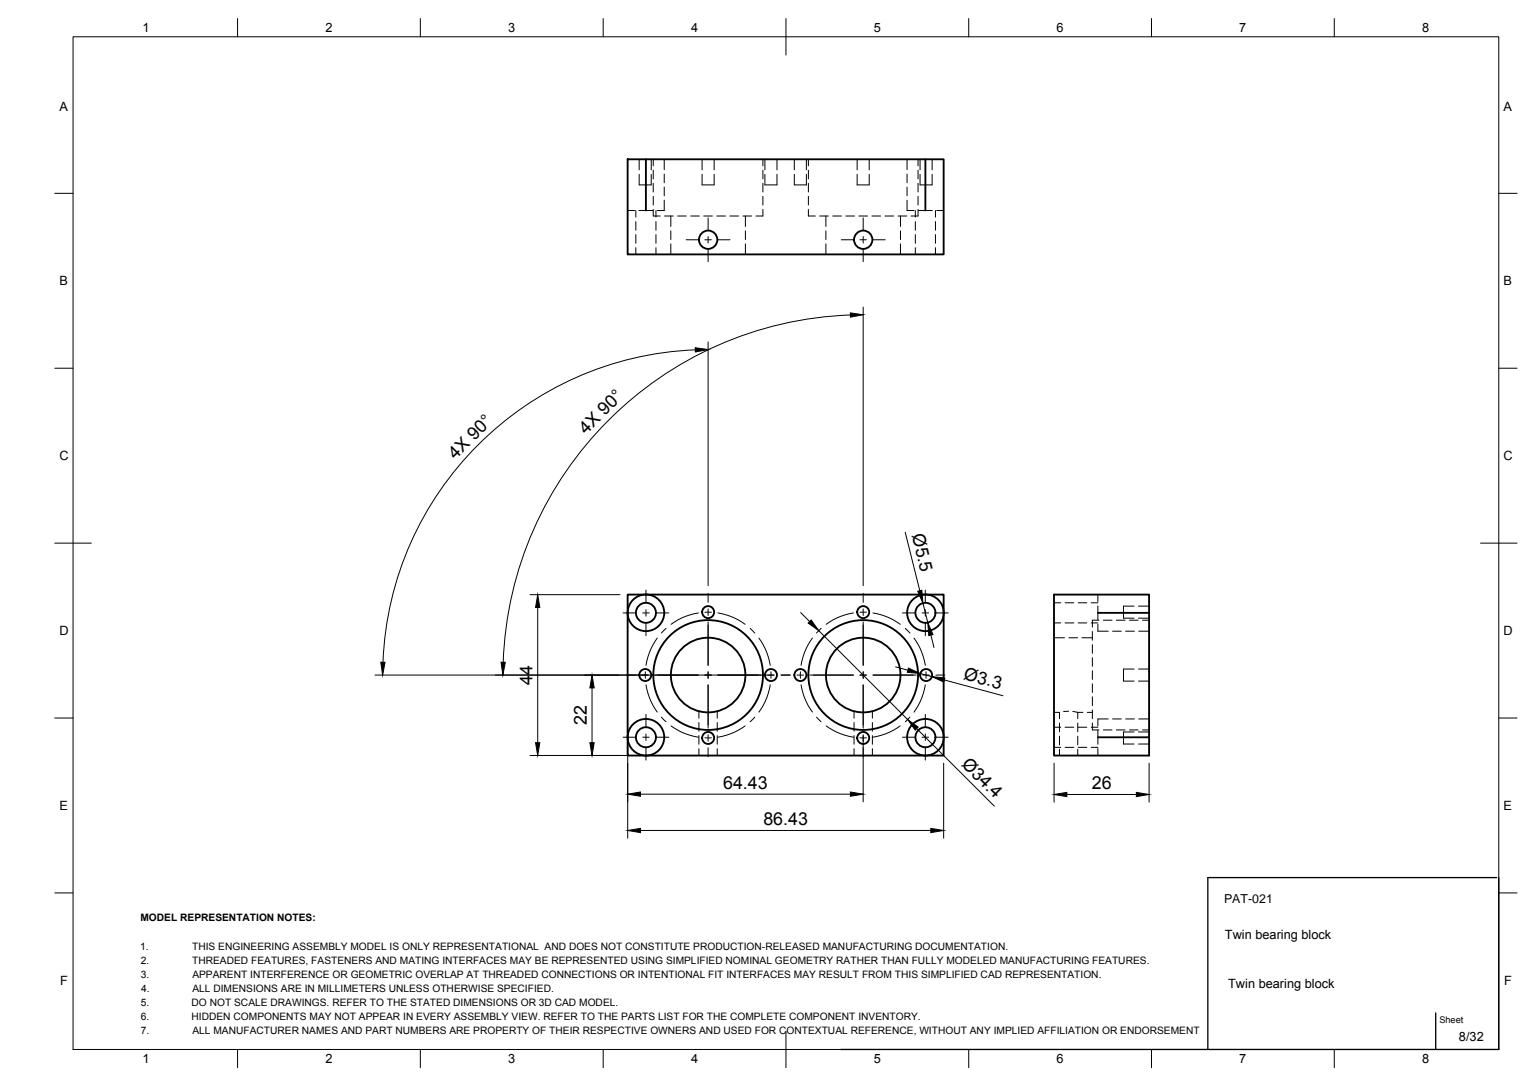
ISO-10303-21;
HEADER;
/* Generated by software containing ST-Developer
 * from STEP Tools, Inc. (www.steptools.com) 
 */

FILE_DESCRIPTION(
/* description */ ('Chain-less indexing wheel (Geneva) drive'),
/* implementation_level */ '2;1');

FILE_NAME(
/* name */ 'Twin bearing block.step',
/* time_stamp */ '2026-10-28T03:25:22-07:00',
/* author */ (''),
/* organization */ (''),
/* preprocessor_version */ 'ST-DEVELOPER v20.2',
/* originating_system */ 'Autodesk Translation Framework v15.17.0.0',
/* authorisation */ '');

FILE_SCHEMA (('AUTOMOTIVE_DESIGN { 1 0 10303 214 3 1 1 }'));
ENDSEC;

DATA;
#10=MECHANICAL_DESIGN_GEOMETRIC_PRESENTATION_REPRESENTATION('',(#306),#10957);
#213=B_SPLINE_CURVE_WITH_KNOTS('',3,(#8714,#8715,#8716,#8717,#8718,#8719,
#8720,#8721,#8722,#8723,#8724,#8725,#8726,#8727,#8728,#8729,#8730,#8731,
#8732,#8733,#8734,#8735,#8736,#8737,#8738,#8739,#8740,#8741,#8742,#8743,
#8744,#8745,#8746,#8747),.UNSPECIFIED.,.T.,.F.,(4,2,2,2,2,2,2,2,2,2,2,2,
2,2,2,2,4),(0.,0.094594182476448,0.189188364952896,0.283770357603024,0.378352350253152,
0.472934342903279,0.567516335553407,0.662110518029855,0.756704700506303,
0.851298882982751,0.945893065459199,1.04047505810933,1.13505705075945,1.22963904340958,
1.32422103605971,1.41881521853616,1.51340940101261),.UNSPECIFIED.);
#214=B_SPLINE_CURVE_WITH_KNOTS('',3,(#8794,#8795,#8796,#8797,#8798,#8799,
#8800,#8801,#8802,#8803,#8804,#8805,#8806,#8807,#8808,#8809,#8810,#8811,
#8812,#8813,#8814,#8815,#8816,#8817,#8818,#8819,#8820,#8821,#8822,#8823,
#8824,#8825,#8826,#8827),.UNSPECIFIED.,.T.,.F.,(4,2,2,2,2,2,2,2,2,2,2,2,
2,2,2,2,4),(0.,0.0945941824764479,0.189188364952896,0.283770357603024,0.378352350253152,
0.47293434290328,0.567516335553408,0.662110518029856,0.756704700506303,
0.851298882982751,0.945893065459199,1.04047505810933,1.13505705075946,1.22963904340958,
1.32422103605971,1.41881521853616,1.51340940101261),.UNSPECIFIED.);
#256=SHAPE_REPRESENTATION_RELATIONSHIP('SRR','None',#11069,#281);
#281=ADVANCED_BREP_SHAPE_REPRESENTATION('',(#339),#10932);
#306=STYLED_ITEM('',(#11287),#339);
#339=MANIFOLD_SOLID_BREP('Body1',#5702);
#375=FACE_BOUND('',#1026,.T.);
#376=FACE_BOUND('',#1028,.T.);
#377=FACE_BOUND('',#1040,.T.);
#378=FACE_BOUND('',#1042,.T.);
#379=FACE_BOUND('',#1046,.T.);
#380=FACE_BOUND('',#1050,.T.);
#381=FACE_BOUND('',#1054,.T.);
#382=FACE_BOUND('',#1058,.T.);
#383=FACE_BOUND('',#1063,.T.);
#384=FACE_BOUND('',#1064,.T.);
#385=FACE_BOUND('',#1065,.T.);
#386=FACE_BOUND('',#1066,.T.);
#387=FACE_BOUND('',#1067,.T.);
#388=FACE_BOUND('',#1068,.T.);
#389=FACE_BOUND('',#1069,.T.);
#390=FACE_BOUND('',#1070,.T.);
#391=FACE_BOUND('',#1071,.T.);
#392=FACE_BOUND('',#1072,.T.);
#393=FACE_BOUND('',#1081,.T.);
#394=FACE_BOUND('',#1082,.T.);
#395=FACE_BOUND('',#1085,.T.);
#396=FACE_BOUND('',#1086,.T.);
#397=FACE_BOUND('',#1087,.T.);
#398=FACE_BOUND('',#1088,.T.);
#399=FACE_BOUND('',#1089,.T.);
#400=FACE_BOUND('',#1090,.T.);
#490=PLANE('',#6051);
#491=PLANE('',#6055);
#492=PLANE('',#6059);
#493=PLANE('',#6063);
#494=PLANE('',#6067);
#495=PLANE('',#6076);
#496=PLANE('',#6080);
#497=PLANE('',#6084);
#498=PLANE('',#6088);
#499=PLANE('',#6092);
#500=PLANE('',#6102);
#501=PLANE('',#6110);
#502=PLANE('',#6118);
#503=PLANE('',#6126);
#504=PLANE('',#6128);
#505=PLANE('',#6129);
#506=PLANE('',#6130);
#507=PLANE('',#6131);
#508=PLANE('',#6132);
#509=PLANE('',#6141);
#510=PLANE('',#6142);
#511=PLANE('',#6143);
#512=PLANE('',#6144);
#513=PLANE('',#6145);
#674=FACE_OUTER_BOUND('',#1015,.T.);
#675=FACE_OUTER_BOUND('',#1016,.T.);
#676=FACE_OUTER_BOUND('',#1017,.T.);
#677=FACE_OUTER_BOUND('',#1018,.T.);
#678=FACE_OUTER_BOUND('',#1019,.T.);
#679=FACE_OUTER_BOUND('',#1020,.T.);
#680=FACE_OUTER_BOUND('',#1021,.T.);
#681=FACE_OUTER_BOUND('',#1022,.T.);
#682=FACE_OUTER_BOUND('',#1023,.T.);
#683=FACE_OUTER_BOUND('',#1024,.T.);
#684=FACE_OUTER_BOUND('',#1025,.T.);
#685=FACE_OUTER_BOUND('',#1027,.T.);
#686=FACE_OUTER_BOUND('',#1029,.T.);
#687=FACE_OUTER_BOUND('',#1030,.T.);
#688=FACE_OUTER_BOUND('',#1031,.T.);
#689=FACE_OUTER_BOUND('',#1032,.T.);
#690=FACE_OUTER_BOUND('',#1033,.T.);
#691=FACE_OUTER_BOUND('',#1034,.T.);
#692=FACE_OUTER_BOUND('',#1035,.T.);
#693=FACE_OUTER_BOUND('',#1036,.T.);
#694=FACE_OUTER_BOUND('',#1037,.T.);
#695=FACE_OUTER_BOUND('',#1038,.T.);
#696=FACE_OUTER_BOUND('',#1039,.T.);
#697=FACE_OUTER_BOUND('',#1041,.T.);
#698=FACE_OUTER_BOUND('',#1043,.T.);
#699=FACE_OUTER_BOUND('',#1044,.T.);
#700=FACE_OUTER_BOUND('',#1045,.T.);
#701=FACE_OUTER_BOUND('',#1047,.T.);
#702=FACE_OUTER_BOUND('',#1048,.T.);
#703=FACE_OUTER_BOUND('',#1049,.T.);
#704=FACE_OUTER_BOUND('',#1051,.T.);
#705=FACE_OUTER_BOUND('',#1052,.T.);
#706=FACE_OUTER_BOUND('',#1053,.T.);
#707=FACE_OUTER_BOUND('',#1055,.T.);
#708=FACE_OUTER_BOUND('',#1056,.T.);
#709=FACE_OUTER_BOUND('',#1057,.T.);
#710=FACE_OUTER_BOUND('',#1059,.T.);
#711=FACE_OUTER_BOUND('',#1060,.T.);
#712=FACE_OUTER_BOUND('',#1061,.T.);
#713=FACE_OUTER_BOUND('',#1062,.T.);
#714=FACE_OUTER_BOUND('',#1073,.T.);
#715=FACE_OUTER_BOUND('',#1074,.T.);
#716=FACE_OUTER_BOUND('',#1075,.T.);
#717=FACE_OUTER_BOUND('',#1076,.T.);
#718=FACE_OUTER_BOUND('',#1077,.T.);
#719=FACE_OUTER_BOUND('',#1078,.T.);
#720=FACE_OUTER_BOUND('',#1079,.T.);
#721=FACE_OUTER_BOUND('',#1080,.T.);
#722=FACE_OUTER_BOUND('',#1083,.T.);
#723=FACE_OUTER_BOUND('',#1084,.T.);
#1015=EDGE_LOOP('',(#3843,#3844,#3845,#3846));
#1016=EDGE_LOOP('',(#3847,#3848,#3849,#3850));
#1017=EDGE_LOOP('',(#3851));
#1018=EDGE_LOOP('',(#3852,#3853,#3854,#3855));
#1019=EDGE_LOOP('',(#3856));
#1020=EDGE_LOOP('',(#3857,#3858,#3859,#3860));
#1021=EDGE_LOOP('',(#3861));
#1022=EDGE_LOOP('',(#3862,#3863,#3864,#3865));
#1023=EDGE_LOOP('',(#3866));
#1024=EDGE_LOOP('',(#3867,#3868,#3869,#3870));
#1025=EDGE_LOOP('',(#3871));
#1026=EDGE_LOOP('',(#3872));
#1027=EDGE_LOOP('',(#3873,#3874,#3875,#3876));
#1028=EDGE_LOOP('',(#3877));
#1029=EDGE_LOOP('',(#3878,#3879,#3880,#3881));
#1030=EDGE_LOOP('',(#3882,#3883,#3884,#3885));
#1031=EDGE_LOOP('',(#3886));
#1032=EDGE_LOOP('',(#3887,#3888,#3889,#3890));
#1033=EDGE_LOOP('',(#3891));
#1034=EDGE_LOOP('',(#3892,#3893,#3894,#3895));
#1035=EDGE_LOOP('',(#3896));
#1036=EDGE_LOOP('',(#3897,#3898,#3899,#3900));
#1037=EDGE_LOOP('',(#3901));
#1038=EDGE_LOOP('',(#3902,#3903,#3904,#3905));
#1039=EDGE_LOOP('',(#3906));
#1040=EDGE_LOOP('',(#3907));
#1041=EDGE_LOOP('',(#3908,#3909,#3910,#3911));
#1042=EDGE_LOOP('',(#3912));
#1043=EDGE_LOOP('',(#3913,#3914,#3915,#3916));
#1044=EDGE_LOOP('',(#3917,#3918,#3919,#3920));
#1045=EDGE_LOOP('',(#3921,#3922));
#1046=EDGE_LOOP('',(#3923));
#1047=EDGE_LOOP('',(#3924,#3925,#3926,#3927));
#1048=EDGE_LOOP('',(#3928,#3929,#3930,#3931));
#1049=EDGE_LOOP('',(#3932,#3933));
#1050=EDGE_LOOP('',(#3934));
#1051=EDGE_LOOP('',(#3935,#3936,#3937,#3938));
#1052=EDGE_LOOP('',(#3939,#3940,#3941,#3942));
#1053=EDGE_LOOP('',(#3943,#3944));
#1054=EDGE_LOOP('',(#3945));
#1055=EDGE_LOOP('',(#3946,#3947,#3948,#3949));
#1056=EDGE_LOOP('',(#3950,#3951,#3952,#3953));
#1057=EDGE_LOOP('',(#3954,#3955));
#1058=EDGE_LOOP('',(#3956));
#1059=EDGE_LOOP('',(#3957,#3958,#3959));
#1060=EDGE_LOOP('',(#3960,#3961,#3962));
#1061=EDGE_LOOP('',(#3963,#3964,#3965));
#1062=EDGE_LOOP('',(#3966,#3967,#3968,#3969,#3970,#3971,#3972,#3973));
#1063=EDGE_LOOP('',(#3974));
#1064=EDGE_LOOP('',(#3975));
#1065=EDGE_LOOP('',(#3976));
#1066=EDGE_LOOP('',(#3977));
#1067=EDGE_LOOP('',(#3978));
#1068=EDGE_LOOP('',(#3979));
#1069=EDGE_LOOP('',(#3980));
#1070=EDGE_LOOP('',(#3981));
#1071=EDGE_LOOP('',(#3982));
#1072=EDGE_LOOP('',(#3983));
#1073=EDGE_LOOP('',(#3984,#3985,#3986));
#1074=EDGE_LOOP('',(#3987,#3988,#3989,#3990));
#1075=EDGE_LOOP('',(#3991,#3992,#3993,#3994));
#1076=EDGE_LOOP('',(#3995,#3996,#3997,#3998));
#1077=EDGE_LOOP('',(#3999,#4000,#4001,#4002));
#1078=EDGE_LOOP('',(#4003,#4004,#4005,#4006,#4007,#4008,#4009,#4010,#4011,
#4012));
#1079=EDGE_LOOP('',(#4013,#4014,#4015,#4016,#4017,#4018,#4019,#4020,#4021,
#4022));
#1080=EDGE_LOOP('',(#4023,#4024,#4025,#4026,#4027,#4028,#4029,#4030,#4031,
#4032));
#1081=EDGE_LOOP('',(#4033));
#1082=EDGE_LOOP('',(#4034));
#1083=EDGE_LOOP('',(#4035,#4036,#4037,#4038,#4039,#4040,#4041,#4042,#4043,
#4044));
#1084=EDGE_LOOP('',(#4045,#4046,#4047,#4048));
#1085=EDGE_LOOP('',(#4049));
#1086=EDGE_LOOP('',(#4050));
#1087=EDGE_LOOP('',(#4051));
#1088=EDGE_LOOP('',(#4052));
#1089=EDGE_LOOP('',(#4053));
#1090=EDGE_LOOP('',(#4054));
#1463=LINE('',#8713,#1837);
#1464=LINE('',#8752,#1838);
#1465=LINE('',#8759,#1839);
#1466=LINE('',#8766,#1840);
#1467=LINE('',#8773,#1841);
#1468=LINE('',#8780,#1842);
#1469=LINE('',#8788,#1843);
#1470=LINE('',#8793,#1844);
#1471=LINE('',#8832,#1845);
#1472=LINE('',#8839,#1846);
#1473=LINE('',#8846,#1847);
#1474=LINE('',#8853,#1848);
#1475=LINE('',#8860,#1849);
#1476=LINE('',#8868,#1850);
#1477=LINE('',#8872,#1851);
#1478=LINE('',#8876,#1852);
#1479=LINE('',#8879,#1853);
#1480=LINE('',#8881,#1854);
#1481=LINE('',#8889,#1855);
#1482=LINE('',#8893,#1856);
#1483=LINE('',#8896,#1857);
#1484=LINE('',#8898,#1858);
#1485=LINE('',#8906,#1859);
#1486=LINE('',#8910,#1860);
#1487=LINE('',#8913,#1861);
#1488=LINE('',#8915,#1862);
#1489=LINE('',#8923,#1863);
#1490=LINE('',#8927,#1864);
#1491=LINE('',#8930,#1865);
#1492=LINE('',#8932,#1866);
#1493=LINE('',#8939,#1867);
#1494=LINE('',#8940,#1868);
#1495=LINE('',#8943,#1869);
#1496=LINE('',#8944,#1870);
#1497=LINE('',#8947,#1871);
#1498=LINE('',#8948,#1872);
#1499=LINE('',#8950,#1873);
#1500=LINE('',#8951,#1874);
#1501=LINE('',#8952,#1875);
#1502=LINE('',#8953,#1876);
#1503=LINE('',#8956,#1877);
#1504=LINE('',#8957,#1878);
#1505=LINE('',#8961,#1879);
#1506=LINE('',#8965,#1880);
#1507=LINE('',#8969,#1881);
#1508=LINE('',#8973,#1882);
#1509=LINE('',#8977,#1883);
#1510=LINE('',#8978,#1884);
#1511=LINE('',#8979,#1885);
#1512=LINE('',#8982,#1886);
#1513=LINE('',#8983,#1887);
#1514=LINE('',#8986,#1888);
#1515=LINE('',#8987,#1889);
#1516=LINE('',#8989,#1890);
#1837=VECTOR('',#6865,0.25);
#1838=VECTOR('',#6870,0.165);
#1839=VECTOR('',#6879,0.165);
#1840=VECTOR('',#6888,0.165);
#1841=VECTOR('',#6897,0.165);
#1842=VECTOR('',#6906,1.5);
#1843=VECTOR('',#6917,1.02);
#1844=VECTOR('',#6922,0.25);
#1845=VECTOR('',#6927,0.165);
#1846=VECTOR('',#6936,0.165);
#1847=VECTOR('',#6945,0.165);
#1848=VECTOR('',#6954,0.165);
#1849=VECTOR('',#6963,1.5);
#1850=VECTOR('',#6974,1.02);
#1851=VECTOR('',#6977,1.);
#1852=VECTOR('',#6980,1.);
#1853=VECTOR('',#6985,1.);
#1854=VECTOR('',#6988,1.);
#1855=VECTOR('',#6997,1.);
#1856=VECTOR('',#7000,1.);
#1857=VECTOR('',#7005,1.);
#1858=VECTOR('',#7008,1.);
#1859=VECTOR('',#7017,1.);
#1860=VECTOR('',#7020,1.);
#1861=VECTOR('',#7025,1.);
#1862=VECTOR('',#7028,1.);
#1863=VECTOR('',#7037,1.);
#1864=VECTOR('',#7040,1.);
#1865=VECTOR('',#7045,1.);
#1866=VECTOR('',#7048,1.);
#1867=VECTOR('',#7057,1.);
#1868=VECTOR('',#7058,1.);
#1869=VECTOR('',#7061,1.);
#1870=VECTOR('',#7062,1.);
#1871=VECTOR('',#7065,1.);
#1872=VECTOR('',#7066,1.);
#1873=VECTOR('',#7069,1.);
#1874=VECTOR('',#7070,1.);
#1875=VECTOR('',#7071,1.);
#1876=VECTOR('',#7072,1.);
#1877=VECTOR('',#7075,1.);
#1878=VECTOR('',#7076,1.);
#1879=VECTOR('',#7081,0.275);
#1880=VECTOR('',#7086,0.275);
#1881=VECTOR('',#7091,0.275);
#1882=VECTOR('',#7096,0.275);
#1883=VECTOR('',#7099,1.);
#1884=VECTOR('',#7100,1.);
#1885=VECTOR('',#7101,1.);
#1886=VECTOR('',#7104,1.);
#1887=VECTOR('',#7105,1.);
#1888=VECTOR('',#7108,1.);
#1889=VECTOR('',#7109,1.);
#1890=VECTOR('',#7112,1.);
#2179=CIRCLE('',#6047,0.25);
#2180=CIRCLE('',#6049,0.165);
#2181=CIRCLE('',#6050,0.165);
#2182=CIRCLE('',#6053,0.165);
#2183=CIRCLE('',#6054,0.165);
#2184=CIRCLE('',#6057,0.165);
#2185=CIRCLE('',#6058,0.165);
#2186=CIRCLE('',#6061,0.165);
#2187=CIRCLE('',#6062,0.165);
#2188=CIRCLE('',#6065,1.5);
#2189=CIRCLE('',#6066,1.5);
#2190=CIRCLE('',#6068,1.02);
#2191=CIRCLE('',#6070,1.02);
#2192=CIRCLE('',#6072,0.25);
#2193=CIRCLE('',#6074,0.165);
#2194=CIRCLE('',#6075,0.165);
#2195=CIRCLE('',#6078,0.165);
#2196=CIRCLE('',#6079,0.165);
#2197=CIRCLE('',#6082,0.165);
#2198=CIRCLE('',#6083,0.165);
#2199=CIRCLE('',#6086,0.165);
#2200=CIRCLE('',#6087,0.165);
#2201=CIRCLE('',#6090,1.5);
#2202=CIRCLE('',#6091,1.5);
#2203=CIRCLE('',#6093,1.02);
#2204=CIRCLE('',#6095,1.02);
#2205=CIRCLE('',#6097,0.5);
#2206=CIRCLE('',#6098,0.5);
#2207=CIRCLE('',#6100,0.5);
#2208=CIRCLE('',#6101,0.5);
#2209=CIRCLE('',#6103,0.275);
#2210=CIRCLE('',#6105,0.5);
#2211=CIRCLE('',#6106,0.5);
#2212=CIRCLE('',#6108,0.5);
#2213=CIRCLE('',#6109,0.5);
#2214=CIRCLE('',#6111,0.275);
#2215=CIRCLE('',#6113,0.5);
#2216=CIRCLE('',#6114,0.5);
#2217=CIRCLE('',#6116,0.5);
#2218=CIRCLE('',#6117,0.5);
#2219=CIRCLE('',#6119,0.275);
#2220=CIRCLE('',#6121,0.5);
#2221=CIRCLE('',#6122,0.5);
#2222=CIRCLE('',#6124,0.5);
#2223=CIRCLE('',#6125,0.5);
#2224=CIRCLE('',#6127,0.275);
#2225=CIRCLE('',#6134,0.275);
#2226=CIRCLE('',#6136,0.275);
#2227=CIRCLE('',#6138,0.275);
#2228=CIRCLE('',#6140,0.275);
#2537=VERTEX_POINT('',#8710);
#2538=VERTEX_POINT('',#8712);
#2539=VERTEX_POINT('',#8749);
#2540=VERTEX_POINT('',#8751);
#2541=VERTEX_POINT('',#8756);
#2542=VERTEX_POINT('',#8758);
#2543=VERTEX_POINT('',#8763);
#2544=VERTEX_POINT('',#8765);
#2545=VERTEX_POINT('',#8770);
#2546=VERTEX_POINT('',#8772);
#2547=VERTEX_POINT('',#8777);
#2548=VERTEX_POINT('',#8779);
#2549=VERTEX_POINT('',#8783);
#2550=VERTEX_POINT('',#8786);
#2551=VERTEX_POINT('',#8790);
#2552=VERTEX_POINT('',#8792);
#2553=VERTEX_POINT('',#8829);
#2554=VERTEX_POINT('',#8831);
#2555=VERTEX_POINT('',#8836);
#2556=VERTEX_POINT('',#8838);
#2557=VERTEX_POINT('',#8843);
#2558=VERTEX_POINT('',#8845);
#2559=VERTEX_POINT('',#8850);
#2560=VERTEX_POINT('',#8852);
#2561=VERTEX_POINT('',#8857);
#2562=VERTEX_POINT('',#8859);
#2563=VERTEX_POINT('',#8863);
#2564=VERTEX_POINT('',#8866);
#2565=VERTEX_POINT('',#8870);
#2566=VERTEX_POINT('',#8871);
#2567=VERTEX_POINT('',#8873);
#2568=VERTEX_POINT('',#8875);
#2569=VERTEX_POINT('',#8884);
#2570=VERTEX_POINT('',#8887);
#2571=VERTEX_POINT('',#8888);
#2572=VERTEX_POINT('',#8890);
#2573=VERTEX_POINT('',#8892);
#2574=VERTEX_POINT('',#8901);
#2575=VERTEX_POINT('',#8904);
#2576=VERTEX_POINT('',#8905);
#2577=VERTEX_POINT('',#8907);
#2578=VERTEX_POINT('',#8909);
#2579=VERTEX_POINT('',#8918);
#2580=VERTEX_POINT('',#8921);
#2581=VERTEX_POINT('',#8922);
#2582=VERTEX_POINT('',#8924);
#2583=VERTEX_POINT('',#8926);
#2584=VERTEX_POINT('',#8935);
#2585=VERTEX_POINT('',#8938);
#2586=VERTEX_POINT('',#8942);
#2587=VERTEX_POINT('',#8946);
#2588=VERTEX_POINT('',#8955);
#2589=VERTEX_POINT('',#8959);
#2590=VERTEX_POINT('',#8963);
#2591=VERTEX_POINT('',#8967);
#2592=VERTEX_POINT('',#8971);
#2593=VERTEX_POINT('',#8975);
#2594=VERTEX_POINT('',#8976);
#2595=VERTEX_POINT('',#8981);
#2596=VERTEX_POINT('',#8985);
#3047=EDGE_CURVE('',#2537,#2537,#2179,.T.);
#3048=EDGE_CURVE('',#2537,#2538,#1463,.T.);
#3049=EDGE_CURVE('',#2538,#2538,#213,.T.);
#3050=EDGE_CURVE('',#2539,#2539,#2180,.T.);
#3051=EDGE_CURVE('',#2539,#2540,#1464,.T.);
#3052=EDGE_CURVE('',#2540,#2540,#2181,.T.);
#3053=EDGE_CURVE('',#2541,#2541,#2182,.T.);
#3054=EDGE_CURVE('',#2541,#2542,#1465,.T.);
#3055=EDGE_CURVE('',#2542,#2542,#2183,.T.);
#3056=EDGE_CURVE('',#2543,#2543,#2184,.T.);
#3057=EDGE_CURVE('',#2543,#2544,#1466,.T.);
#3058=EDGE_CURVE('',#2544,#2544,#2185,.T.);
#3059=EDGE_CURVE('',#2545,#2545,#2186,.T.);
#3060=EDGE_CURVE('',#2545,#2546,#1467,.T.);
#3061=EDGE_CURVE('',#2546,#2546,#2187,.T.);
#3062=EDGE_CURVE('',#2547,#2547,#2188,.T.);
#3063=EDGE_CURVE('',#2547,#2548,#1468,.T.);
#3064=EDGE_CURVE('',#2548,#2548,#2189,.T.);
#3065=EDGE_CURVE('',#2549,#2549,#2190,.T.);
#3066=EDGE_CURVE('',#2550,#2550,#2191,.T.);
#3067=EDGE_CURVE('',#2550,#2549,#1469,.T.);
#3068=EDGE_CURVE('',#2551,#2551,#2192,.T.);
#3069=EDGE_CURVE('',#2551,#2552,#1470,.T.);
#3070=EDGE_CURVE('',#2552,#2552,#214,.T.);
#3071=EDGE_CURVE('',#2553,#2553,#2193,.T.);
#3072=EDGE_CURVE('',#2553,#2554,#1471,.T.);
#3073=EDGE_CURVE('',#2554,#2554,#2194,.T.);
#3074=EDGE_CURVE('',#2555,#2555,#2195,.T.);
#3075=EDGE_CURVE('',#2555,#2556,#1472,.T.);
#3076=EDGE_CURVE('',#2556,#2556,#2196,.T.);
#3077=EDGE_CURVE('',#2557,#2557,#2197,.T.);
#3078=EDGE_CURVE('',#2557,#2558,#1473,.T.);
#3079=EDGE_CURVE('',#2558,#2558,#2198,.T.);
#3080=EDGE_CURVE('',#2559,#2559,#2199,.T.);
#3081=EDGE_CURVE('',#2559,#2560,#1474,.T.);
#3082=EDGE_CURVE('',#2560,#2560,#2200,.T.);
#3083=EDGE_CURVE('',#2561,#2561,#2201,.T.);
#3084=EDGE_CURVE('',#2561,#2562,#1475,.T.);
#3085=EDGE_CURVE('',#2562,#2562,#2202,.T.);
#3086=EDGE_CURVE('',#2563,#2563,#2203,.T.);
#3087=EDGE_CURVE('',#2564,#2564,#2204,.T.);
#3088=EDGE_CURVE('',#2564,#2563,#1476,.T.);
#3089=EDGE_CURVE('',#2565,#2566,#1477,.T.);
#3090=EDGE_CURVE('',#2567,#2566,#2205,.T.);
#3091=EDGE_CURVE('',#2568,#2567,#1478,.T.);
#3092=EDGE_CURVE('',#2565,#2568,#2206,.T.);
#3093=EDGE_CURVE('',#2565,#2566,#1479,.T.);
#3094=EDGE_CURVE('',#2568,#2565,#2207,.T.);
#3095=EDGE_CURVE('',#2568,#2567,#1480,.T.);
#3096=EDGE_CURVE('',#2566,#2567,#2208,.T.);
#3097=EDGE_CURVE('',#2569,#2569,#2209,.T.);
#3098=EDGE_CURVE('',#2570,#2571,#1481,.T.);
#3099=EDGE_CURVE('',#2572,#2571,#2210,.T.);
#3100=EDGE_CURVE('',#2573,#2572,#1482,.T.);
#3101=EDGE_CURVE('',#2570,#2573,#2211,.T.);
#3102=EDGE_CURVE('',#2570,#2571,#1483,.T.);
#3103=EDGE_CURVE('',#2573,#2570,#2212,.T.);
#3104=EDGE_CURVE('',#2573,#2572,#1484,.T.);
#3105=EDGE_CURVE('',#2571,#2572,#2213,.T.);
#3106=EDGE_CURVE('',#2574,#2574,#2214,.T.);
#3107=EDGE_CURVE('',#2575,#2576,#1485,.T.);
#3108=EDGE_CURVE('',#2577,#2576,#2215,.T.);
#3109=EDGE_CURVE('',#2578,#2577,#1486,.T.);
#3110=EDGE_CURVE('',#2575,#2578,#2216,.T.);
#3111=EDGE_CURVE('',#2575,#2576,#1487,.T.);
#3112=EDGE_CURVE('',#2578,#2575,#2217,.T.);
#3113=EDGE_CURVE('',#2578,#2577,#1488,.T.);
#3114=EDGE_CURVE('',#2576,#2577,#2218,.T.);
#3115=EDGE_CURVE('',#2579,#2579,#2219,.T.);
#3116=EDGE_CURVE('',#2580,#2581,#1489,.T.);
#3117=EDGE_CURVE('',#2582,#2581,#2220,.T.);
#3118=EDGE_CURVE('',#2583,#2582,#1490,.T.);
#3119=EDGE_CURVE('',#2580,#2583,#2221,.T.);
#3120=EDGE_CURVE('',#2580,#2581,#1491,.T.);
#3121=EDGE_CURVE('',#2583,#2580,#2222,.T.);
#3122=EDGE_CURVE('',#2583,#2582,#1492,.T.);
#3123=EDGE_CURVE('',#2581,#2582,#2223,.T.);
#3124=EDGE_CURVE('',#2584,#2584,#2224,.T.);
#3125=EDGE_CURVE('',#2582,#2585,#1493,.T.);
#3126=EDGE_CURVE('',#2585,#2581,#1494,.T.);
#3127=EDGE_CURVE('',#2577,#2586,#1495,.T.);
#3128=EDGE_CURVE('',#2586,#2576,#1496,.T.);
#3129=EDGE_CURVE('',#2571,#2587,#1497,.T.);
#3130=EDGE_CURVE('',#2587,#2572,#1498,.T.);
#3131=EDGE_CURVE('',#2566,#2582,#1499,.T.);
#3132=EDGE_CURVE('',#2581,#2571,#1500,.T.);
#3133=EDGE_CURVE('',#2572,#2577,#1501,.T.);
#3134=EDGE_CURVE('',#2576,#2567,#1502,.T.);
#3135=EDGE_CURVE('',#2567,#2588,#1503,.T.);
#3136=EDGE_CURVE('',#2588,#2566,#1504,.T.);
#3137=EDGE_CURVE('',#2589,#2589,#2225,.T.);
#3138=EDGE_CURVE('',#2589,#2569,#1505,.T.);
#3139=EDGE_CURVE('',#2590,#2590,#2226,.T.);
#3140=EDGE_CURVE('',#2590,#2574,#1506,.T.);
#3141=EDGE_CURVE('',#2591,#2591,#2227,.T.);
#3142=EDGE_CURVE('',#2591,#2579,#1507,.T.);
#3143=EDGE_CURVE('',#2592,#2592,#2228,.T.);
#3144=EDGE_CURVE('',#2592,#2584,#1508,.T.);
#3145=EDGE_CURVE('',#2593,#2594,#1509,.T.);
#3146=EDGE_CURVE('',#2594,#2587,#1510,.T.);
#3147=EDGE_CURVE('',#2593,#2585,#1511,.T.);
#3148=EDGE_CURVE('',#2595,#2593,#1512,.T.);
#3149=EDGE_CURVE('',#2595,#2588,#1513,.T.);
#3150=EDGE_CURVE('',#2596,#2595,#1514,.T.);
#3151=EDGE_CURVE('',#2596,#2586,#1515,.T.);
#3152=EDGE_CURVE('',#2594,#2596,#1516,.T.);
#3843=ORIENTED_EDGE('',*,*,#3047,.F.);
#3844=ORIENTED_EDGE('',*,*,#3048,.T.);
#3845=ORIENTED_EDGE('',*,*,#3049,.F.);
#3846=ORIENTED_EDGE('',*,*,#3048,.F.);
#3847=ORIENTED_EDGE('',*,*,#3050,.F.);
#3848=ORIENTED_EDGE('',*,*,#3051,.T.);
#3849=ORIENTED_EDGE('',*,*,#3052,.F.);
#3850=ORIENTED_EDGE('',*,*,#3051,.F.);
#3851=ORIENTED_EDGE('',*,*,#3050,.T.);
#3852=ORIENTED_EDGE('',*,*,#3053,.F.);
#3853=ORIENTED_EDGE('',*,*,#3054,.T.);
#3854=ORIENTED_EDGE('',*,*,#3055,.F.);
#3855=ORIENTED_EDGE('',*,*,#3054,.F.);
#3856=ORIENTED_EDGE('',*,*,#3053,.T.);
#3857=ORIENTED_EDGE('',*,*,#3056,.F.);
#3858=ORIENTED_EDGE('',*,*,#3057,.T.);
#3859=ORIENTED_EDGE('',*,*,#3058,.F.);
#3860=ORIENTED_EDGE('',*,*,#3057,.F.);
#3861=ORIENTED_EDGE('',*,*,#3056,.T.);
#3862=ORIENTED_EDGE('',*,*,#3059,.F.);
#3863=ORIENTED_EDGE('',*,*,#3060,.T.);
#3864=ORIENTED_EDGE('',*,*,#3061,.F.);
#3865=ORIENTED_EDGE('',*,*,#3060,.F.);
#3866=ORIENTED_EDGE('',*,*,#3059,.T.);
#3867=ORIENTED_EDGE('',*,*,#3062,.F.);
#3868=ORIENTED_EDGE('',*,*,#3063,.T.);
#3869=ORIENTED_EDGE('',*,*,#3064,.F.);
#3870=ORIENTED_EDGE('',*,*,#3063,.F.);
#3871=ORIENTED_EDGE('',*,*,#3062,.T.);
#3872=ORIENTED_EDGE('',*,*,#3065,.F.);
#3873=ORIENTED_EDGE('',*,*,#3066,.F.);
#3874=ORIENTED_EDGE('',*,*,#3067,.T.);
#3875=ORIENTED_EDGE('',*,*,#3065,.T.);
#3876=ORIENTED_EDGE('',*,*,#3067,.F.);
#3877=ORIENTED_EDGE('',*,*,#3049,.T.);
#3878=ORIENTED_EDGE('',*,*,#3068,.F.);
#3879=ORIENTED_EDGE('',*,*,#3069,.T.);
#3880=ORIENTED_EDGE('',*,*,#3070,.F.);
#3881=ORIENTED_EDGE('',*,*,#3069,.F.);
#3882=ORIENTED_EDGE('',*,*,#3071,.F.);
#3883=ORIENTED_EDGE('',*,*,#3072,.T.);
#3884=ORIENTED_EDGE('',*,*,#3073,.F.);
#3885=ORIENTED_EDGE('',*,*,#3072,.F.);
#3886=ORIENTED_EDGE('',*,*,#3071,.T.);
#3887=ORIENTED_EDGE('',*,*,#3074,.F.);
#3888=ORIENTED_EDGE('',*,*,#3075,.T.);
#3889=ORIENTED_EDGE('',*,*,#3076,.F.);
#3890=ORIENTED_EDGE('',*,*,#3075,.F.);
#3891=ORIENTED_EDGE('',*,*,#3074,.T.);
#3892=ORIENTED_EDGE('',*,*,#3077,.F.);
#3893=ORIENTED_EDGE('',*,*,#3078,.T.);
#3894=ORIENTED_EDGE('',*,*,#3079,.F.);
#3895=ORIENTED_EDGE('',*,*,#3078,.F.);
#3896=ORIENTED_EDGE('',*,*,#3077,.T.);
#3897=ORIENTED_EDGE('',*,*,#3080,.F.);
#3898=ORIENTED_EDGE('',*,*,#3081,.T.);
#3899=ORIENTED_EDGE('',*,*,#3082,.F.);
#3900=ORIENTED_EDGE('',*,*,#3081,.F.);
#3901=ORIENTED_EDGE('',*,*,#3080,.T.);
#3902=ORIENTED_EDGE('',*,*,#3083,.F.);
#3903=ORIENTED_EDGE('',*,*,#3084,.T.);
#3904=ORIENTED_EDGE('',*,*,#3085,.F.);
#3905=ORIENTED_EDGE('',*,*,#3084,.F.);
#3906=ORIENTED_EDGE('',*,*,#3083,.T.);
#3907=ORIENTED_EDGE('',*,*,#3086,.F.);
#3908=ORIENTED_EDGE('',*,*,#3087,.F.);
#3909=ORIENTED_EDGE('',*,*,#3088,.T.);
#3910=ORIENTED_EDGE('',*,*,#3086,.T.);
#3911=ORIENTED_EDGE('',*,*,#3088,.F.);
#3912=ORIENTED_EDGE('',*,*,#3070,.T.);
#3913=ORIENTED_EDGE('',*,*,#3089,.T.);
#3914=ORIENTED_EDGE('',*,*,#3090,.F.);
#3915=ORIENTED_EDGE('',*,*,#3091,.F.);
#3916=ORIENTED_EDGE('',*,*,#3092,.F.);
#3917=ORIENTED_EDGE('',*,*,#3093,.F.);
#3918=ORIENTED_EDGE('',*,*,#3094,.F.);
#3919=ORIENTED_EDGE('',*,*,#3095,.T.);
#3920=ORIENTED_EDGE('',*,*,#3096,.F.);
#3921=ORIENTED_EDGE('',*,*,#3092,.T.);
#3922=ORIENTED_EDGE('',*,*,#3094,.T.);
#3923=ORIENTED_EDGE('',*,*,#3097,.F.);
#3924=ORIENTED_EDGE('',*,*,#3098,.T.);
#3925=ORIENTED_EDGE('',*,*,#3099,.F.);
#3926=ORIENTED_EDGE('',*,*,#3100,.F.);
#3927=ORIENTED_EDGE('',*,*,#3101,.F.);
#3928=ORIENTED_EDGE('',*,*,#3102,.F.);
#3929=ORIENTED_EDGE('',*,*,#3103,.F.);
#3930=ORIENTED_EDGE('',*,*,#3104,.T.);
#3931=ORIENTED_EDGE('',*,*,#3105,.F.);
#3932=ORIENTED_EDGE('',*,*,#3103,.T.);
#3933=ORIENTED_EDGE('',*,*,#3101,.T.);
#3934=ORIENTED_EDGE('',*,*,#3106,.F.);
#3935=ORIENTED_EDGE('',*,*,#3107,.T.);
#3936=ORIENTED_EDGE('',*,*,#3108,.F.);
#3937=ORIENTED_EDGE('',*,*,#3109,.F.);
#3938=ORIENTED_EDGE('',*,*,#3110,.F.);
#3939=ORIENTED_EDGE('',*,*,#3111,.F.);
#3940=ORIENTED_EDGE('',*,*,#3112,.F.);
#3941=ORIENTED_EDGE('',*,*,#3113,.T.);
#3942=ORIENTED_EDGE('',*,*,#3114,.F.);
#3943=ORIENTED_EDGE('',*,*,#3112,.T.);
#3944=ORIENTED_EDGE('',*,*,#3110,.T.);
#3945=ORIENTED_EDGE('',*,*,#3115,.F.);
#3946=ORIENTED_EDGE('',*,*,#3116,.T.);
#3947=ORIENTED_EDGE('',*,*,#3117,.F.);
#3948=ORIENTED_EDGE('',*,*,#3118,.F.);
#3949=ORIENTED_EDGE('',*,*,#3119,.F.);
#3950=ORIENTED_EDGE('',*,*,#3120,.F.);
#3951=ORIENTED_EDGE('',*,*,#3121,.F.);
#3952=ORIENTED_EDGE('',*,*,#3122,.T.);
#3953=ORIENTED_EDGE('',*,*,#3123,.F.);
#3954=ORIENTED_EDGE('',*,*,#3119,.T.);
#3955=ORIENTED_EDGE('',*,*,#3121,.T.);
#3956=ORIENTED_EDGE('',*,*,#3124,.F.);
#3957=ORIENTED_EDGE('',*,*,#3123,.T.);
#3958=ORIENTED_EDGE('',*,*,#3125,.T.);
#3959=ORIENTED_EDGE('',*,*,#3126,.T.);
#3960=ORIENTED_EDGE('',*,*,#3114,.T.);
#3961=ORIENTED_EDGE('',*,*,#3127,.T.);
#3962=ORIENTED_EDGE('',*,*,#3128,.T.);
#3963=ORIENTED_EDGE('',*,*,#3099,.T.);
#3964=ORIENTED_EDGE('',*,*,#3129,.T.);
#3965=ORIENTED_EDGE('',*,*,#3130,.T.);
#3966=ORIENTED_EDGE('',*,*,#3090,.T.);
#3967=ORIENTED_EDGE('',*,*,#3131,.T.);
#3968=ORIENTED_EDGE('',*,*,#3117,.T.);
#3969=ORIENTED_EDGE('',*,*,#3132,.T.);
#3970=ORIENTED_EDGE('',*,*,#3105,.T.);
#3971=ORIENTED_EDGE('',*,*,#3133,.T.);
#3972=ORIENTED_EDGE('',*,*,#3108,.T.);
#3973=ORIENTED_EDGE('',*,*,#3134,.T.);
#3974=ORIENTED_EDGE('',*,*,#3073,.T.);
#3975=ORIENTED_EDGE('',*,*,#3076,.T.);
#3976=ORIENTED_EDGE('',*,*,#3079,.T.);
#3977=ORIENTED_EDGE('',*,*,#3082,.T.);
#3978=ORIENTED_EDGE('',*,*,#3085,.T.);
#3979=ORIENTED_EDGE('',*,*,#3064,.T.);
#3980=ORIENTED_EDGE('',*,*,#3061,.T.);
#3981=ORIENTED_EDGE('',*,*,#3058,.T.);
#3982=ORIENTED_EDGE('',*,*,#3055,.T.);
#3983=ORIENTED_EDGE('',*,*,#3052,.T.);
#3984=ORIENTED_EDGE('',*,*,#3096,.T.);
#3985=ORIENTED_EDGE('',*,*,#3135,.T.);
#3986=ORIENTED_EDGE('',*,*,#3136,.T.);
#3987=ORIENTED_EDGE('',*,*,#3137,.F.);
#3988=ORIENTED_EDGE('',*,*,#3138,.T.);
#3989=ORIENTED_EDGE('',*,*,#3097,.T.);
#3990=ORIENTED_EDGE('',*,*,#3138,.F.);
#3991=ORIENTED_EDGE('',*,*,#3139,.F.);
#3992=ORIENTED_EDGE('',*,*,#3140,.T.);
#3993=ORIENTED_EDGE('',*,*,#3106,.T.);
#3994=ORIENTED_EDGE('',*,*,#3140,.F.);
#3995=ORIENTED_EDGE('',*,*,#3141,.F.);
#3996=ORIENTED_EDGE('',*,*,#3142,.T.);
#3997=ORIENTED_EDGE('',*,*,#3115,.T.);
#3998=ORIENTED_EDGE('',*,*,#3142,.F.);
#3999=ORIENTED_EDGE('',*,*,#3143,.F.);
#4000=ORIENTED_EDGE('',*,*,#3144,.T.);
#4001=ORIENTED_EDGE('',*,*,#3124,.T.);
#4002=ORIENTED_EDGE('',*,*,#3144,.F.);
#4003=ORIENTED_EDGE('',*,*,#3145,.T.);
#4004=ORIENTED_EDGE('',*,*,#3146,.T.);
#4005=ORIENTED_EDGE('',*,*,#3129,.F.);
#4006=ORIENTED_EDGE('',*,*,#3098,.F.);
#4007=ORIENTED_EDGE('',*,*,#3102,.T.);
#4008=ORIENTED_EDGE('',*,*,#3132,.F.);
#4009=ORIENTED_EDGE('',*,*,#3116,.F.);
#4010=ORIENTED_EDGE('',*,*,#3120,.T.);
#4011=ORIENTED_EDGE('',*,*,#3126,.F.);
#4012=ORIENTED_EDGE('',*,*,#3147,.F.);
#4013=ORIENTED_EDGE('',*,*,#3148,.T.);
#4014=ORIENTED_EDGE('',*,*,#3147,.T.);
#4015=ORIENTED_EDGE('',*,*,#3125,.F.);
#4016=ORIENTED_EDGE('',*,*,#3122,.F.);
#4017=ORIENTED_EDGE('',*,*,#3118,.T.);
#4018=ORIENTED_EDGE('',*,*,#3131,.F.);
#4019=ORIENTED_EDGE('',*,*,#3089,.F.);
#4020=ORIENTED_EDGE('',*,*,#3093,.T.);
#4021=ORIENTED_EDGE('',*,*,#3136,.F.);
#4022=ORIENTED_EDGE('',*,*,#3149,.F.);
#4023=ORIENTED_EDGE('',*,*,#3150,.T.);
#4024=ORIENTED_EDGE('',*,*,#3149,.T.);
#4025=ORIENTED_EDGE('',*,*,#3135,.F.);
#4026=ORIENTED_EDGE('',*,*,#3095,.F.);
#4027=ORIENTED_EDGE('',*,*,#3091,.T.);
#4028=ORIENTED_EDGE('',*,*,#3134,.F.);
#4029=ORIENTED_EDGE('',*,*,#3107,.F.);
#4030=ORIENTED_EDGE('',*,*,#3111,.T.);
#4031=ORIENTED_EDGE('',*,*,#3128,.F.);
#4032=ORIENTED_EDGE('',*,*,#3151,.F.);
#4033=ORIENTED_EDGE('',*,*,#3047,.T.);
#4034=ORIENTED_EDGE('',*,*,#3068,.T.);
#4035=ORIENTED_EDGE('',*,*,#3152,.T.);
#4036=ORIENTED_EDGE('',*,*,#3151,.T.);
#4037=ORIENTED_EDGE('',*,*,#3127,.F.);
#4038=ORIENTED_EDGE('',*,*,#3113,.F.);
#4039=ORIENTED_EDGE('',*,*,#3109,.T.);
#4040=ORIENTED_EDGE('',*,*,#3133,.F.);
#4041=ORIENTED_EDGE('',*,*,#3104,.F.);
#4042=ORIENTED_EDGE('',*,*,#3100,.T.);
#4043=ORIENTED_EDGE('',*,*,#3130,.F.);
#4044=ORIENTED_EDGE('',*,*,#3146,.F.);
#4045=ORIENTED_EDGE('',*,*,#3152,.F.);
#4046=ORIENTED_EDGE('',*,*,#3145,.F.);
#4047=ORIENTED_EDGE('',*,*,#3148,.F.);
#4048=ORIENTED_EDGE('',*,*,#3150,.F.);
#4049=ORIENTED_EDGE('',*,*,#3066,.T.);
#4050=ORIENTED_EDGE('',*,*,#3087,.T.);
#4051=ORIENTED_EDGE('',*,*,#3137,.T.);
#4052=ORIENTED_EDGE('',*,*,#3139,.T.);
#4053=ORIENTED_EDGE('',*,*,#3141,.T.);
#4054=ORIENTED_EDGE('',*,*,#3143,.T.);
#5247=CYLINDRICAL_SURFACE('',#6046,0.25);
#5248=CYLINDRICAL_SURFACE('',#6048,0.165);
#5249=CYLINDRICAL_SURFACE('',#6052,0.165);
#5250=CYLINDRICAL_SURFACE('',#6056,0.165);
#5251=CYLINDRICAL_SURFACE('',#6060,0.165);
#5252=CYLINDRICAL_SURFACE('',#6064,1.5);
#5253=CYLINDRICAL_SURFACE('',#6069,1.02);
#5254=CYLINDRICAL_SURFACE('',#6071,0.25);
#5255=CYLINDRICAL_SURFACE('',#6073,0.165);
#5256=CYLINDRICAL_SURFACE('',#6077,0.165);
#5257=CYLINDRICAL_SURFACE('',#6081,0.165);
#5258=CYLINDRICAL_SURFACE('',#6085,0.165);
#5259=CYLINDRICAL_SURFACE('',#6089,1.5);
#5260=CYLINDRICAL_SURFACE('',#6094,1.02);
#5261=CYLINDRICAL_SURFACE('',#6096,0.5);
#5262=CYLINDRICAL_SURFACE('',#6099,0.5);
#5263=CYLINDRICAL_SURFACE('',#6104,0.5);
#5264=CYLINDRICAL_SURFACE('',#6107,0.5);
#5265=CYLINDRICAL_SURFACE('',#6112,0.5);
#5266=CYLINDRICAL_SURFACE('',#6115,0.5);
#5267=CYLINDRICAL_SURFACE('',#6120,0.5);
#5268=CYLINDRICAL_SURFACE('',#6123,0.5);
#5269=CYLINDRICAL_SURFACE('',#6133,0.275);
#5270=CYLINDRICAL_SURFACE('',#6135,0.275);
#5271=CYLINDRICAL_SURFACE('',#6137,0.275);
#5272=CYLINDRICAL_SURFACE('',#6139,0.275);
#5388=ADVANCED_FACE('',(#674),#5247,.F.);
#5389=ADVANCED_FACE('',(#675),#5248,.F.);
#5390=ADVANCED_FACE('',(#676),#490,.T.);
#5391=ADVANCED_FACE('',(#677),#5249,.F.);
#5392=ADVANCED_FACE('',(#678),#491,.T.);
#5393=ADVANCED_FACE('',(#679),#5250,.F.);
#5394=ADVANCED_FACE('',(#680),#492,.T.);
#5395=ADVANCED_FACE('',(#681),#5251,.F.);
#5396=ADVANCED_FACE('',(#682),#493,.T.);
#5397=ADVANCED_FACE('',(#683),#5252,.F.);
#5398=ADVANCED_FACE('',(#684,#375),#494,.T.);
#5399=ADVANCED_FACE('',(#685,#376),#5253,.F.);
#5400=ADVANCED_FACE('',(#686),#5254,.F.);
#5401=ADVANCED_FACE('',(#687),#5255,.F.);
#5402=ADVANCED_FACE('',(#688),#495,.T.);
#5403=ADVANCED_FACE('',(#689),#5256,.F.);
#5404=ADVANCED_FACE('',(#690),#496,.T.);
#5405=ADVANCED_FACE('',(#691),#5257,.F.);
#5406=ADVANCED_FACE('',(#692),#497,.T.);
#5407=ADVANCED_FACE('',(#693),#5258,.F.);
#5408=ADVANCED_FACE('',(#694),#498,.T.);
#5409=ADVANCED_FACE('',(#695),#5259,.F.);
#5410=ADVANCED_FACE('',(#696,#377),#499,.T.);
#5411=ADVANCED_FACE('',(#697,#378),#5260,.F.);
#5412=ADVANCED_FACE('',(#698),#5261,.F.);
#5413=ADVANCED_FACE('',(#699),#5262,.F.);
#5414=ADVANCED_FACE('',(#700,#379),#500,.T.);
#5415=ADVANCED_FACE('',(#701),#5263,.F.);
#5416=ADVANCED_FACE('',(#702),#5264,.F.);
#5417=ADVANCED_FACE('',(#703,#380),#501,.T.);
#5418=ADVANCED_FACE('',(#704),#5265,.F.);
#5419=ADVANCED_FACE('',(#705),#5266,.F.);
#5420=ADVANCED_FACE('',(#706,#381),#502,.T.);
#5421=ADVANCED_FACE('',(#707),#5267,.F.);
#5422=ADVANCED_FACE('',(#708),#5268,.F.);
#5423=ADVANCED_FACE('',(#709,#382),#503,.T.);
#5424=ADVANCED_FACE('',(#710),#504,.T.);
#5425=ADVANCED_FACE('',(#711),#505,.T.);
#5426=ADVANCED_FACE('',(#712),#506,.T.);
#5427=ADVANCED_FACE('',(#713,#383,#384,#385,#386,#387,#388,#389,#390,#391,
#392),#507,.T.);
#5428=ADVANCED_FACE('',(#714),#508,.T.);
#5429=ADVANCED_FACE('',(#715),#5269,.F.);
#5430=ADVANCED_FACE('',(#716),#5270,.F.);
#5431=ADVANCED_FACE('',(#717),#5271,.F.);
#5432=ADVANCED_FACE('',(#718),#5272,.F.);
#5433=ADVANCED_FACE('',(#719),#509,.T.);
#5434=ADVANCED_FACE('',(#720),#510,.T.);
#5435=ADVANCED_FACE('',(#721,#393,#394),#511,.T.);
#5436=ADVANCED_FACE('',(#722),#512,.T.);
#5437=ADVANCED_FACE('',(#723,#395,#396,#397,#398,#399,#400),#513,.F.);
#5702=CLOSED_SHELL('',(#5388,#5389,#5390,#5391,#5392,#5393,#5394,#5395,
#5396,#5397,#5398,#5399,#5400,#5401,#5402,#5403,#5404,#5405,#5406,#5407,
#5408,#5409,#5410,#5411,#5412,#5413,#5414,#5415,#5416,#5417,#5418,#5419,
#5420,#5421,#5422,#5423,#5424,#5425,#5426,#5427,#5428,#5429,#5430,#5431,
#5432,#5433,#5434,#5435,#5436,#5437));
#6045=AXIS2_PLACEMENT_3D('',#8708,#6859,#6860);
#6046=AXIS2_PLACEMENT_3D('',#8709,#6861,#6862);
#6047=AXIS2_PLACEMENT_3D('',#8711,#6863,#6864);
#6048=AXIS2_PLACEMENT_3D('',#8748,#6866,#6867);
#6049=AXIS2_PLACEMENT_3D('',#8750,#6868,#6869);
#6050=AXIS2_PLACEMENT_3D('',#8753,#6871,#6872);
#6051=AXIS2_PLACEMENT_3D('',#8754,#6873,#6874);
#6052=AXIS2_PLACEMENT_3D('',#8755,#6875,#6876);
#6053=AXIS2_PLACEMENT_3D('',#8757,#6877,#6878);
#6054=AXIS2_PLACEMENT_3D('',#8760,#6880,#6881);
#6055=AXIS2_PLACEMENT_3D('',#8761,#6882,#6883);
#6056=AXIS2_PLACEMENT_3D('',#8762,#6884,#6885);
#6057=AXIS2_PLACEMENT_3D('',#8764,#6886,#6887);
#6058=AXIS2_PLACEMENT_3D('',#8767,#6889,#6890);
#6059=AXIS2_PLACEMENT_3D('',#8768,#6891,#6892);
#6060=AXIS2_PLACEMENT_3D('',#8769,#6893,#6894);
#6061=AXIS2_PLACEMENT_3D('',#8771,#6895,#6896);
#6062=AXIS2_PLACEMENT_3D('',#8774,#6898,#6899);
#6063=AXIS2_PLACEMENT_3D('',#8775,#6900,#6901);
#6064=AXIS2_PLACEMENT_3D('',#8776,#6902,#6903);
#6065=AXIS2_PLACEMENT_3D('',#8778,#6904,#6905);
#6066=AXIS2_PLACEMENT_3D('',#8781,#6907,#6908);
#6067=AXIS2_PLACEMENT_3D('',#8782,#6909,#6910);
#6068=AXIS2_PLACEMENT_3D('',#8784,#6911,#6912);
#6069=AXIS2_PLACEMENT_3D('',#8785,#6913,#6914);
#6070=AXIS2_PLACEMENT_3D('',#8787,#6915,#6916);
#6071=AXIS2_PLACEMENT_3D('',#8789,#6918,#6919);
#6072=AXIS2_PLACEMENT_3D('',#8791,#6920,#6921);
#6073=AXIS2_PLACEMENT_3D('',#8828,#6923,#6924);
#6074=AXIS2_PLACEMENT_3D('',#8830,#6925,#6926);
#6075=AXIS2_PLACEMENT_3D('',#8833,#6928,#6929);
#6076=AXIS2_PLACEMENT_3D('',#8834,#6930,#6931);
#6077=AXIS2_PLACEMENT_3D('',#8835,#6932,#6933);
#6078=AXIS2_PLACEMENT_3D('',#8837,#6934,#6935);
#6079=AXIS2_PLACEMENT_3D('',#8840,#6937,#6938);
#6080=AXIS2_PLACEMENT_3D('',#8841,#6939,#6940);
#6081=AXIS2_PLACEMENT_3D('',#8842,#6941,#6942);
#6082=AXIS2_PLACEMENT_3D('',#8844,#6943,#6944);
#6083=AXIS2_PLACEMENT_3D('',#8847,#6946,#6947);
#6084=AXIS2_PLACEMENT_3D('',#8848,#6948,#6949);
#6085=AXIS2_PLACEMENT_3D('',#8849,#6950,#6951);
#6086=AXIS2_PLACEMENT_3D('',#8851,#6952,#6953);
#6087=AXIS2_PLACEMENT_3D('',#8854,#6955,#6956);
#6088=AXIS2_PLACEMENT_3D('',#8855,#6957,#6958);
#6089=AXIS2_PLACEMENT_3D('',#8856,#6959,#6960);
#6090=AXIS2_PLACEMENT_3D('',#8858,#6961,#6962);
#6091=AXIS2_PLACEMENT_3D('',#8861,#6964,#6965);
#6092=AXIS2_PLACEMENT_3D('',#8862,#6966,#6967);
#6093=AXIS2_PLACEMENT_3D('',#8864,#6968,#6969);
#6094=AXIS2_PLACEMENT_3D('',#8865,#6970,#6971);
#6095=AXIS2_PLACEMENT_3D('',#8867,#6972,#6973);
#6096=AXIS2_PLACEMENT_3D('',#8869,#6975,#6976);
#6097=AXIS2_PLACEMENT_3D('',#8874,#6978,#6979);
#6098=AXIS2_PLACEMENT_3D('',#8877,#6981,#6982);
#6099=AXIS2_PLACEMENT_3D('',#8878,#6983,#6984);
#6100=AXIS2_PLACEMENT_3D('',#8880,#6986,#6987);
#6101=AXIS2_PLACEMENT_3D('',#8882,#6989,#6990);
#6102=AXIS2_PLACEMENT_3D('',#8883,#6991,#6992);
#6103=AXIS2_PLACEMENT_3D('',#8885,#6993,#6994);
#6104=AXIS2_PLACEMENT_3D('',#8886,#6995,#6996);
#6105=AXIS2_PLACEMENT_3D('',#8891,#6998,#6999);
#6106=AXIS2_PLACEMENT_3D('',#8894,#7001,#7002);
#6107=AXIS2_PLACEMENT_3D('',#8895,#7003,#7004);
#6108=AXIS2_PLACEMENT_3D('',#8897,#7006,#7007);
#6109=AXIS2_PLACEMENT_3D('',#8899,#7009,#7010);
#6110=AXIS2_PLACEMENT_3D('',#8900,#7011,#7012);
#6111=AXIS2_PLACEMENT_3D('',#8902,#7013,#7014);
#6112=AXIS2_PLACEMENT_3D('',#8903,#7015,#7016);
#6113=AXIS2_PLACEMENT_3D('',#8908,#7018,#7019);
#6114=AXIS2_PLACEMENT_3D('',#8911,#7021,#7022);
#6115=AXIS2_PLACEMENT_3D('',#8912,#7023,#7024);
#6116=AXIS2_PLACEMENT_3D('',#8914,#7026,#7027);
#6117=AXIS2_PLACEMENT_3D('',#8916,#7029,#7030);
#6118=AXIS2_PLACEMENT_3D('',#8917,#7031,#7032);
#6119=AXIS2_PLACEMENT_3D('',#8919,#7033,#7034);
#6120=AXIS2_PLACEMENT_3D('',#8920,#7035,#7036);
#6121=AXIS2_PLACEMENT_3D('',#8925,#7038,#7039);
#6122=AXIS2_PLACEMENT_3D('',#8928,#7041,#7042);
#6123=AXIS2_PLACEMENT_3D('',#8929,#7043,#7044);
#6124=AXIS2_PLACEMENT_3D('',#8931,#7046,#7047);
#6125=AXIS2_PLACEMENT_3D('',#8933,#7049,#7050);
#6126=AXIS2_PLACEMENT_3D('',#8934,#7051,#7052);
#6127=AXIS2_PLACEMENT_3D('',#8936,#7053,#7054);
#6128=AXIS2_PLACEMENT_3D('',#8937,#7055,#7056);
#6129=AXIS2_PLACEMENT_3D('',#8941,#7059,#7060);
#6130=AXIS2_PLACEMENT_3D('',#8945,#7063,#7064);
#6131=AXIS2_PLACEMENT_3D('',#8949,#7067,#7068);
#6132=AXIS2_PLACEMENT_3D('',#8954,#7073,#7074);
#6133=AXIS2_PLACEMENT_3D('',#8958,#7077,#7078);
#6134=AXIS2_PLACEMENT_3D('',#8960,#7079,#7080);
#6135=AXIS2_PLACEMENT_3D('',#8962,#7082,#7083);
#6136=AXIS2_PLACEMENT_3D('',#8964,#7084,#7085);
#6137=AXIS2_PLACEMENT_3D('',#8966,#7087,#7088);
#6138=AXIS2_PLACEMENT_3D('',#8968,#7089,#7090);
#6139=AXIS2_PLACEMENT_3D('',#8970,#7092,#7093);
#6140=AXIS2_PLACEMENT_3D('',#8972,#7094,#7095);
#6141=AXIS2_PLACEMENT_3D('',#8974,#7097,#7098);
#6142=AXIS2_PLACEMENT_3D('',#8980,#7102,#7103);
#6143=AXIS2_PLACEMENT_3D('',#8984,#7106,#7107);
#6144=AXIS2_PLACEMENT_3D('',#8988,#7110,#7111);
#6145=AXIS2_PLACEMENT_3D('',#8990,#7113,#7114);
#6859=DIRECTION('axis',(0.,0.,1.));
#6860=DIRECTION('refdir',(1.,0.,0.));
#6861=DIRECTION('center_axis',(0.,1.,0.));
#6862=DIRECTION('ref_axis',(1.,0.,0.));
#6863=DIRECTION('center_axis',(0.,1.,0.));
#6864=DIRECTION('ref_axis',(1.,0.,0.));
#6865=DIRECTION('',(0.,1.,0.));
#6866=DIRECTION('center_axis',(0.,0.,1.));
#6867=DIRECTION('ref_axis',(1.,0.,0.));
#6868=DIRECTION('center_axis',(0.,0.,1.));
#6869=DIRECTION('ref_axis',(1.,0.,0.));
#6870=DIRECTION('',(0.,0.,1.));
#6871=DIRECTION('center_axis',(0.,0.,-1.));
#6872=DIRECTION('ref_axis',(1.,0.,0.));
#6873=DIRECTION('center_axis',(0.,0.,1.));
#6874=DIRECTION('ref_axis',(1.,0.,0.));
#6875=DIRECTION('center_axis',(0.,0.,1.));
#6876=DIRECTION('ref_axis',(1.,0.,0.));
#6877=DIRECTION('center_axis',(0.,0.,1.));
#6878=DIRECTION('ref_axis',(1.,0.,0.));
#6879=DIRECTION('',(0.,0.,1.));
#6880=DIRECTION('center_axis',(0.,0.,-1.));
#6881=DIRECTION('ref_axis',(1.,0.,0.));
#6882=DIRECTION('center_axis',(0.,0.,1.));
#6883=DIRECTION('ref_axis',(1.,0.,0.));
#6884=DIRECTION('center_axis',(0.,0.,1.));
#6885=DIRECTION('ref_axis',(1.,0.,0.));
#6886=DIRECTION('center_axis',(0.,0.,1.));
#6887=DIRECTION('ref_axis',(1.,0.,0.));
#6888=DIRECTION('',(0.,0.,1.));
#6889=DIRECTION('center_axis',(0.,0.,-1.));
#6890=DIRECTION('ref_axis',(1.,0.,0.));
#6891=DIRECTION('center_axis',(0.,0.,1.));
#6892=DIRECTION('ref_axis',(1.,0.,0.));
#6893=DIRECTION('center_axis',(0.,0.,1.));
#6894=DIRECTION('ref_axis',(1.,0.,0.));
#6895=DIRECTION('center_axis',(0.,0.,1.));
#6896=DIRECTION('ref_axis',(1.,0.,0.));
#6897=DIRECTION('',(0.,0.,1.));
#6898=DIRECTION('center_axis',(0.,0.,-1.));
#6899=DIRECTION('ref_axis',(1.,0.,0.));
#6900=DIRECTION('center_axis',(0.,0.,1.));
#6901=DIRECTION('ref_axis',(1.,0.,0.));
#6902=DIRECTION('center_axis',(0.,0.,1.));
#6903=DIRECTION('ref_axis',(1.,0.,0.));
#6904=DIRECTION('center_axis',(0.,0.,1.));
#6905=DIRECTION('ref_axis',(1.,0.,0.));
#6906=DIRECTION('',(0.,0.,1.));
#6907=DIRECTION('center_axis',(0.,0.,-1.));
#6908=DIRECTION('ref_axis',(1.,0.,0.));
#6909=DIRECTION('center_axis',(0.,0.,1.));
#6910=DIRECTION('ref_axis',(1.,0.,0.));
#6911=DIRECTION('center_axis',(0.,0.,1.));
#6912=DIRECTION('ref_axis',(1.,0.,0.));
#6913=DIRECTION('center_axis',(0.,0.,1.));
#6914=DIRECTION('ref_axis',(1.,0.,0.));
#6915=DIRECTION('center_axis',(0.,0.,1.));
#6916=DIRECTION('ref_axis',(1.,0.,0.));
#6917=DIRECTION('',(0.,0.,1.));
#6918=DIRECTION('center_axis',(0.,1.,0.));
#6919=DIRECTION('ref_axis',(1.,0.,0.));
#6920=DIRECTION('center_axis',(0.,1.,0.));
#6921=DIRECTION('ref_axis',(1.,0.,0.));
#6922=DIRECTION('',(0.,1.,0.));
#6923=DIRECTION('center_axis',(0.,0.,1.));
#6924=DIRECTION('ref_axis',(1.,0.,0.));
#6925=DIRECTION('center_axis',(0.,0.,1.));
#6926=DIRECTION('ref_axis',(1.,0.,0.));
#6927=DIRECTION('',(0.,0.,1.));
#6928=DIRECTION('center_axis',(0.,0.,-1.));
#6929=DIRECTION('ref_axis',(1.,0.,0.));
#6930=DIRECTION('center_axis',(0.,0.,1.));
#6931=DIRECTION('ref_axis',(1.,0.,0.));
#6932=DIRECTION('center_axis',(0.,0.,1.));
#6933=DIRECTION('ref_axis',(1.,0.,0.));
#6934=DIRECTION('center_axis',(0.,0.,1.));
#6935=DIRECTION('ref_axis',(1.,0.,0.));
#6936=DIRECTION('',(0.,0.,1.));
#6937=DIRECTION('center_axis',(0.,0.,-1.));
#6938=DIRECTION('ref_axis',(1.,0.,0.));
#6939=DIRECTION('center_axis',(0.,0.,1.));
#6940=DIRECTION('ref_axis',(1.,0.,0.));
#6941=DIRECTION('center_axis',(0.,0.,1.));
#6942=DIRECTION('ref_axis',(1.,0.,0.));
#6943=DIRECTION('center_axis',(0.,0.,1.));
#6944=DIRECTION('ref_axis',(1.,0.,0.));
#6945=DIRECTION('',(0.,0.,1.));
#6946=DIRECTION('center_axis',(0.,0.,-1.));
#6947=DIRECTION('ref_axis',(1.,0.,0.));
#6948=DIRECTION('center_axis',(0.,0.,1.));
#6949=DIRECTION('ref_axis',(1.,0.,0.));
#6950=DIRECTION('center_axis',(0.,0.,1.));
#6951=DIRECTION('ref_axis',(1.,0.,0.));
#6952=DIRECTION('center_axis',(0.,0.,1.));
#6953=DIRECTION('ref_axis',(1.,0.,0.));
#6954=DIRECTION('',(0.,0.,1.));
#6955=DIRECTION('center_axis',(0.,0.,-1.));
#6956=DIRECTION('ref_axis',(1.,0.,0.));
#6957=DIRECTION('center_axis',(0.,0.,1.));
#6958=DIRECTION('ref_axis',(1.,0.,0.));
#6959=DIRECTION('center_axis',(0.,0.,1.));
#6960=DIRECTION('ref_axis',(1.,0.,0.));
#6961=DIRECTION('center_axis',(0.,0.,1.));
#6962=DIRECTION('ref_axis',(1.,0.,0.));
#6963=DIRECTION('',(0.,0.,1.));
#6964=DIRECTION('center_axis',(0.,0.,-1.));
#6965=DIRECTION('ref_axis',(1.,0.,0.));
#6966=DIRECTION('center_axis',(0.,0.,1.));
#6967=DIRECTION('ref_axis',(1.,0.,0.));
#6968=DIRECTION('center_axis',(0.,0.,1.));
#6969=DIRECTION('ref_axis',(1.,0.,0.));
#6970=DIRECTION('center_axis',(0.,0.,1.));
#6971=DIRECTION('ref_axis',(1.,0.,0.));
#6972=DIRECTION('center_axis',(0.,0.,1.));
#6973=DIRECTION('ref_axis',(1.,0.,0.));
#6974=DIRECTION('',(0.,0.,1.));
#6975=DIRECTION('center_axis',(0.,0.,1.));
#6976=DIRECTION('ref_axis',(-0.707106781186547,0.707106781186548,0.));
#6977=DIRECTION('',(0.,0.,1.));
#6978=DIRECTION('center_axis',(0.,0.,-1.));
#6979=DIRECTION('ref_axis',(1.,0.,0.));
#6980=DIRECTION('',(0.,0.,1.));
#6981=DIRECTION('center_axis',(0.,0.,1.));
#6982=DIRECTION('ref_axis',(1.,0.,0.));
#6983=DIRECTION('center_axis',(0.,0.,1.));
#6984=DIRECTION('ref_axis',(1.,0.,0.));
#6985=DIRECTION('',(0.,0.,1.));
#6986=DIRECTION('center_axis',(0.,0.,1.));
#6987=DIRECTION('ref_axis',(1.,0.,0.));
#6988=DIRECTION('',(0.,0.,1.));
#6989=DIRECTION('center_axis',(0.,0.,-1.));
#6990=DIRECTION('ref_axis',(1.,0.,0.));
#6991=DIRECTION('center_axis',(0.,0.,1.));
#6992=DIRECTION('ref_axis',(1.,0.,0.));
#6993=DIRECTION('center_axis',(0.,0.,1.));
#6994=DIRECTION('ref_axis',(1.,0.,0.));
#6995=DIRECTION('center_axis',(0.,0.,1.));
#6996=DIRECTION('ref_axis',(1.,0.,0.));
#6997=DIRECTION('',(0.,0.,1.));
#6998=DIRECTION('center_axis',(0.,0.,-1.));
#6999=DIRECTION('ref_axis',(1.,0.,0.));
#7000=DIRECTION('',(0.,0.,1.));
#7001=DIRECTION('center_axis',(0.,0.,1.));
#7002=DIRECTION('ref_axis',(1.,0.,0.));
#7003=DIRECTION('center_axis',(0.,0.,1.));
#7004=DIRECTION('ref_axis',(1.,0.,0.));
#7005=DIRECTION('',(0.,0.,1.));
#7006=DIRECTION('center_axis',(0.,0.,1.));
#7007=DIRECTION('ref_axis',(1.,0.,0.));
#7008=DIRECTION('',(0.,0.,1.));
#7009=DIRECTION('center_axis',(0.,0.,-1.));
#7010=DIRECTION('ref_axis',(1.,0.,0.));
#7011=DIRECTION('center_axis',(0.,0.,1.));
#7012=DIRECTION('ref_axis',(1.,0.,0.));
#7013=DIRECTION('center_axis',(0.,0.,1.));
#7014=DIRECTION('ref_axis',(1.,0.,0.));
#7015=DIRECTION('center_axis',(0.,0.,1.));
#7016=DIRECTION('ref_axis',(1.,0.,0.));
#7017=DIRECTION('',(0.,0.,1.));
#7018=DIRECTION('center_axis',(0.,0.,-1.));
#7019=DIRECTION('ref_axis',(1.,0.,0.));
#7020=DIRECTION('',(0.,0.,1.));
#7021=DIRECTION('center_axis',(0.,0.,1.));
#7022=DIRECTION('ref_axis',(1.,0.,0.));
#7023=DIRECTION('center_axis',(0.,0.,1.));
#7024=DIRECTION('ref_axis',(1.,0.,0.));
#7025=DIRECTION('',(0.,0.,1.));
#7026=DIRECTION('center_axis',(0.,0.,1.));
#7027=DIRECTION('ref_axis',(1.,0.,0.));
#7028=DIRECTION('',(0.,0.,1.));
#7029=DIRECTION('center_axis',(0.,0.,-1.));
#7030=DIRECTION('ref_axis',(1.,0.,0.));
#7031=DIRECTION('center_axis',(0.,0.,1.));
#7032=DIRECTION('ref_axis',(1.,0.,0.));
#7033=DIRECTION('center_axis',(0.,0.,1.));
#7034=DIRECTION('ref_axis',(1.,0.,0.));
#7035=DIRECTION('center_axis',(0.,0.,1.));
#7036=DIRECTION('ref_axis',(-0.707106781186548,-0.707106781186547,0.));
#7037=DIRECTION('',(0.,0.,1.));
#7038=DIRECTION('center_axis',(0.,0.,-1.));
#7039=DIRECTION('ref_axis',(1.,0.,0.));
#7040=DIRECTION('',(0.,0.,1.));
#7041=DIRECTION('center_axis',(0.,0.,1.));
#7042=DIRECTION('ref_axis',(1.,0.,0.));
#7043=DIRECTION('center_axis',(0.,0.,1.));
#7044=DIRECTION('ref_axis',(1.,0.,0.));
#7045=DIRECTION('',(0.,0.,1.));
#7046=DIRECTION('center_axis',(0.,0.,1.));
#7047=DIRECTION('ref_axis',(1.,0.,0.));
#7048=DIRECTION('',(0.,0.,1.));
#7049=DIRECTION('center_axis',(0.,0.,-1.));
#7050=DIRECTION('ref_axis',(1.,0.,0.));
#7051=DIRECTION('center_axis',(0.,0.,1.));
#7052=DIRECTION('ref_axis',(1.,0.,0.));
#7053=DIRECTION('center_axis',(0.,0.,1.));
#7054=DIRECTION('ref_axis',(1.,0.,0.));
#7055=DIRECTION('center_axis',(0.,0.,1.));
#7056=DIRECTION('ref_axis',(1.,0.,0.));
#7057=DIRECTION('',(0.,1.,0.));
#7058=DIRECTION('',(-1.,0.,0.));
#7059=DIRECTION('center_axis',(0.,0.,1.));
#7060=DIRECTION('ref_axis',(1.,0.,0.));
#7061=DIRECTION('',(0.,-1.,0.));
#7062=DIRECTION('',(1.,0.,0.));
#7063=DIRECTION('center_axis',(0.,0.,1.));
#7064=DIRECTION('ref_axis',(1.,0.,0.));
#7065=DIRECTION('',(-1.,0.,0.));
#7066=DIRECTION('',(0.,-1.,0.));
#7067=DIRECTION('center_axis',(0.,0.,1.));
#7068=DIRECTION('ref_axis',(1.,0.,0.));
#7069=DIRECTION('',(0.,1.,0.));
#7070=DIRECTION('',(-1.,0.,0.));
#7071=DIRECTION('',(0.,-1.,0.));
#7072=DIRECTION('',(1.,0.,0.));
#7073=DIRECTION('center_axis',(0.,0.,1.));
#7074=DIRECTION('ref_axis',(1.,0.,0.));
#7075=DIRECTION('',(1.,0.,0.));
#7076=DIRECTION('',(0.,1.,0.));
#7077=DIRECTION('center_axis',(0.,0.,1.));
#7078=DIRECTION('ref_axis',(1.,0.,0.));
#7079=DIRECTION('center_axis',(0.,0.,1.));
#7080=DIRECTION('ref_axis',(1.,0.,0.));
#7081=DIRECTION('',(0.,0.,1.));
#7082=DIRECTION('center_axis',(0.,0.,1.));
#7083=DIRECTION('ref_axis',(1.,0.,0.));
#7084=DIRECTION('center_axis',(0.,0.,1.));
#7085=DIRECTION('ref_axis',(1.,0.,0.));
#7086=DIRECTION('',(0.,0.,1.));
#7087=DIRECTION('center_axis',(0.,0.,1.));
#7088=DIRECTION('ref_axis',(1.,0.,0.));
#7089=DIRECTION('center_axis',(0.,0.,1.));
#7090=DIRECTION('ref_axis',(1.,0.,0.));
#7091=DIRECTION('',(0.,0.,1.));
#7092=DIRECTION('center_axis',(0.,0.,1.));
#7093=DIRECTION('ref_axis',(1.,0.,0.));
#7094=DIRECTION('center_axis',(0.,0.,1.));
#7095=DIRECTION('ref_axis',(1.,0.,0.));
#7096=DIRECTION('',(0.,0.,1.));
#7097=DIRECTION('center_axis',(0.,1.,0.));
#7098=DIRECTION('ref_axis',(-1.,0.,0.));
#7099=DIRECTION('',(-1.,0.,0.));
#7100=DIRECTION('',(0.,0.,1.));
#7101=DIRECTION('',(0.,0.,1.));
#7102=DIRECTION('center_axis',(1.,0.,0.));
#7103=DIRECTION('ref_axis',(0.,1.,0.));
#7104=DIRECTION('',(0.,1.,0.));
#7105=DIRECTION('',(0.,0.,1.));
#7106=DIRECTION('center_axis',(0.,-1.,0.));
#7107=DIRECTION('ref_axis',(1.,0.,0.));
#7108=DIRECTION('',(1.,0.,0.));
#7109=DIRECTION('',(0.,0.,1.));
#7110=DIRECTION('center_axis',(-1.,0.,0.));
#7111=DIRECTION('ref_axis',(0.,-1.,0.));
#7112=DIRECTION('',(0.,-1.,0.));
#7113=DIRECTION('center_axis',(0.,0.,1.));
#7114=DIRECTION('ref_axis',(1.,0.,0.));
#8708=CARTESIAN_POINT('',(0.,0.,0.));
#8709=CARTESIAN_POINT('Origin',(4.24264068711929,-2.3,1.4));
#8710=CARTESIAN_POINT('',(3.99264068711929,-2.2,1.4));
#8711=CARTESIAN_POINT('Origin',(4.24264068711929,-2.2,1.4));
#8712=CARTESIAN_POINT('',(3.99264068711929,-0.988888264668966,1.4));
#8713=CARTESIAN_POINT('',(3.99264068711929,-2.3,1.4));
#8714=CARTESIAN_POINT('Ctrl Pts',(3.99264068711929,-0.988888264668966,1.4));
#8715=CARTESIAN_POINT('Ctrl Pts',(3.99264068711929,-0.988888264668966,1.36846860584118));
#8716=CARTESIAN_POINT('Ctrl Pts',(3.99896863868788,-0.990553370646674,1.33492785033683));
#8717=CARTESIAN_POINT('Ctrl Pts',(4.02452085710491,-0.996491737296663,1.27337379025046));
#8718=CARTESIAN_POINT('Ctrl Pts',(4.04373855891321,-1.00067109353237,1.2453487376128));
#8719=CARTESIAN_POINT('Ctrl Pts',(4.08798657355057,-1.00845756932386,1.20110072297544));
#8720=CARTESIAN_POINT('Ctrl Pts',(4.11601281617403,-1.01258144235289,1.18188079690607));
#8721=CARTESIAN_POINT('Ctrl Pts',(4.17757108672792,-1.0183917429657,1.15632695599232));
#8722=CARTESIAN_POINT('Ctrl Pts',(4.21111335623591,-1.02,1.15));
#8723=CARTESIAN_POINT('Ctrl Pts',(4.27416801800266,-1.02,1.15));
#8724=CARTESIAN_POINT('Ctrl Pts',(4.30771028751065,-1.0183917429657,1.15632695599232));
#8725=CARTESIAN_POINT('Ctrl Pts',(4.36926855806454,-1.01258144235289,1.18188079690607));
#8726=CARTESIAN_POINT('Ctrl Pts',(4.397294800688,-1.00845756932386,1.20110072297544));
#8727=CARTESIAN_POINT('Ctrl Pts',(4.44154281532536,-1.00067109353237,1.2453487376128));
#8728=CARTESIAN_POINT('Ctrl Pts',(4.46076051713366,-0.996491737296663,1.27337379025046));
#8729=CARTESIAN_POINT('Ctrl Pts',(4.48631273555069,-0.990553370646674,1.33492785033683));
#8730=CARTESIAN_POINT('Ctrl Pts',(4.49264068711929,-0.988888264668966,1.36846860584118));
#8731=CARTESIAN_POINT('Ctrl Pts',(4.49264068711929,-0.988888264668966,1.43153139415882));
#8732=CARTESIAN_POINT('Ctrl Pts',(4.48631273555069,-0.990553370646674,1.46507214966317));
#8733=CARTESIAN_POINT('Ctrl Pts',(4.46076051713366,-0.996491737296663,1.52662620974954));
#8734=CARTESIAN_POINT('Ctrl Pts',(4.44154281532536,-1.00067109353237,1.5546512623872));
#8735=CARTESIAN_POINT('Ctrl Pts',(4.397294800688,-1.00845756932386,1.59889927702456));
#8736=CARTESIAN_POINT('Ctrl Pts',(4.36926855806454,-1.01258144235289,1.61811920309393));
#8737=CARTESIAN_POINT('Ctrl Pts',(4.30771028751065,-1.0183917429657,1.64367304400768));
#8738=CARTESIAN_POINT('Ctrl Pts',(4.27416801800266,-1.02,1.65));
#8739=CARTESIAN_POINT('Ctrl Pts',(4.21111335623591,-1.02,1.65));
#8740=CARTESIAN_POINT('Ctrl Pts',(4.17757108672792,-1.0183917429657,1.64367304400768));
#8741=CARTESIAN_POINT('Ctrl Pts',(4.11601281617403,-1.01258144235289,1.61811920309393));
#8742=CARTESIAN_POINT('Ctrl Pts',(4.08798657355057,-1.00845756932386,1.59889927702456));
#8743=CARTESIAN_POINT('Ctrl Pts',(4.04373855891321,-1.00067109353237,1.5546512623872));
#8744=CARTESIAN_POINT('Ctrl Pts',(4.02452085710491,-0.996491737296663,1.52662620974954));
#8745=CARTESIAN_POINT('Ctrl Pts',(3.99896863868788,-0.990553370646674,1.46507214966317));
#8746=CARTESIAN_POINT('Ctrl Pts',(3.99264068711929,-0.988888264668966,1.43153139415882));
#8747=CARTESIAN_POINT('Ctrl Pts',(3.99264068711929,-0.988888264668966,1.4));
#8748=CARTESIAN_POINT('Origin',(2.52264068711929,2.10639249453345E-16,2.9));
#8749=CARTESIAN_POINT('',(2.35764068711929,1.90432577267413E-16,2.9));
#8750=CARTESIAN_POINT('Origin',(2.52264068711929,2.10639249453345E-16,2.9));
#8751=CARTESIAN_POINT('',(2.35764068711929,2.30845921639276E-16,3.6));
#8752=CARTESIAN_POINT('',(2.35764068711929,1.90432577267413E-16,2.9));
#8753=CARTESIAN_POINT('Origin',(2.52264068711929,2.10639249453345E-16,3.6));
#8754=CARTESIAN_POINT('Origin',(2.52264068711929,2.22044604925031E-16,2.9));
#8755=CARTESIAN_POINT('Origin',(4.24264068711929,1.72,2.9));
#8756=CARTESIAN_POINT('',(4.07764068711929,1.72,2.9));
#8757=CARTESIAN_POINT('Origin',(4.24264068711929,1.72,2.9));
#8758=CARTESIAN_POINT('',(4.07764068711929,1.72,3.6));
#8759=CARTESIAN_POINT('',(4.07764068711929,1.72,2.9));
#8760=CARTESIAN_POINT('Origin',(4.24264068711929,1.72,3.6));
#8761=CARTESIAN_POINT('Origin',(4.24264068711929,1.72,2.9));
#8762=CARTESIAN_POINT('Origin',(5.96264068711929,0.,2.9));
#8763=CARTESIAN_POINT('',(5.79764068711929,-2.02066721859313E-17,2.9));
#8764=CARTESIAN_POINT('Origin',(5.96264068711929,0.,2.9));
#8765=CARTESIAN_POINT('',(5.79764068711929,2.02066721859313E-17,3.6));
#8766=CARTESIAN_POINT('',(5.79764068711929,-2.02066721859313E-17,2.9));
#8767=CARTESIAN_POINT('Origin',(5.96264068711929,0.,3.6));
#8768=CARTESIAN_POINT('Origin',(5.96264068711929,0.,2.9));
#8769=CARTESIAN_POINT('Origin',(4.24264068711929,-1.72,2.9));
#8770=CARTESIAN_POINT('',(4.07764068711929,-1.72,2.9));
#8771=CARTESIAN_POINT('Origin',(4.24264068711929,-1.72,2.9));
#8772=CARTESIAN_POINT('',(4.07764068711929,-1.72,3.6));
#8773=CARTESIAN_POINT('',(4.07764068711929,-1.72,2.9));
#8774=CARTESIAN_POINT('Origin',(4.24264068711929,-1.72,3.6));
#8775=CARTESIAN_POINT('Origin',(4.24264068711929,-1.72,2.9));
#8776=CARTESIAN_POINT('Origin',(4.24264068711929,0.,2.05));
#8777=CARTESIAN_POINT('',(2.74264068711929,-1.83697019872103E-16,2.05));
#8778=CARTESIAN_POINT('Origin',(4.24264068711929,0.,2.05));
#8779=CARTESIAN_POINT('',(2.74264068711929,1.83697019872103E-16,3.6));
#8780=CARTESIAN_POINT('',(2.74264068711929,-1.83697019872103E-16,2.05));
#8781=CARTESIAN_POINT('Origin',(4.24264068711929,0.,3.6));
#8782=CARTESIAN_POINT('Origin',(4.24264068711929,0.,2.05));
#8783=CARTESIAN_POINT('',(3.22264068711929,-1.2491397351303E-16,2.05));
#8784=CARTESIAN_POINT('Origin',(4.24264068711929,0.,2.05));
#8785=CARTESIAN_POINT('Origin',(4.24264068711929,0.,0.9));
#8786=CARTESIAN_POINT('',(3.22264068711929,-1.2491397351303E-16,1.));
#8787=CARTESIAN_POINT('Origin',(4.24264068711929,0.,1.));
#8788=CARTESIAN_POINT('',(3.22264068711929,-1.2491397351303E-16,0.9));
#8789=CARTESIAN_POINT('Origin',(0.,-2.3,1.4));
#8790=CARTESIAN_POINT('',(-0.25,-2.2,1.4));
#8791=CARTESIAN_POINT('Origin',(0.,-2.2,1.4));
#8792=CARTESIAN_POINT('',(-0.25,-0.988888264668967,1.4));
#8793=CARTESIAN_POINT('',(-0.25,-2.3,1.4));
#8794=CARTESIAN_POINT('Ctrl Pts',(-0.25,-0.988888264668967,1.4));
#8795=CARTESIAN_POINT('Ctrl Pts',(-0.25,-0.988888264668967,1.36846860584118));
#8796=CARTESIAN_POINT('Ctrl Pts',(-0.243672048431404,-0.990553370646674,
1.33492785033683));
#8797=CARTESIAN_POINT('Ctrl Pts',(-0.218119830014375,-0.996491737296663,
1.27337379025046));
#8798=CARTESIAN_POINT('Ctrl Pts',(-0.198902128206072,-1.00067109353237,
1.2453487376128));
#8799=CARTESIAN_POINT('Ctrl Pts',(-0.154654113568716,-1.00845756932386,
1.20110072297544));
#8800=CARTESIAN_POINT('Ctrl Pts',(-0.126627870945253,-1.01258144235289,
1.18188079690607));
#8801=CARTESIAN_POINT('Ctrl Pts',(-0.0650696003913631,-1.0183917429657,
1.15632695599232));
#8802=CARTESIAN_POINT('Ctrl Pts',(-0.031527330883376,-1.02,1.15));
#8803=CARTESIAN_POINT('Ctrl Pts',(0.031527330883376,-1.02,1.15));
#8804=CARTESIAN_POINT('Ctrl Pts',(0.065069600391363,-1.0183917429657,1.15632695599232));
#8805=CARTESIAN_POINT('Ctrl Pts',(0.126627870945253,-1.01258144235289,1.18188079690607));
#8806=CARTESIAN_POINT('Ctrl Pts',(0.154654113568716,-1.00845756932386,1.20110072297544));
#8807=CARTESIAN_POINT('Ctrl Pts',(0.198902128206072,-1.00067109353237,1.2453487376128));
#8808=CARTESIAN_POINT('Ctrl Pts',(0.218119830014375,-0.996491737296663,
1.27337379025046));
#8809=CARTESIAN_POINT('Ctrl Pts',(0.243672048431404,-0.990553370646674,
1.33492785033683));
#8810=CARTESIAN_POINT('Ctrl Pts',(0.25,-0.988888264668967,1.36846860584118));
#8811=CARTESIAN_POINT('Ctrl Pts',(0.25,-0.988888264668967,1.43153139415882));
#8812=CARTESIAN_POINT('Ctrl Pts',(0.243672048431404,-0.990553370646674,
1.46507214966317));
#8813=CARTESIAN_POINT('Ctrl Pts',(0.218119830014375,-0.996491737296663,
1.52662620974954));
#8814=CARTESIAN_POINT('Ctrl Pts',(0.198902128206072,-1.00067109353237,1.5546512623872));
#8815=CARTESIAN_POINT('Ctrl Pts',(0.154654113568716,-1.00845756932386,1.59889927702456));
#8816=CARTESIAN_POINT('Ctrl Pts',(0.126627870945253,-1.01258144235289,1.61811920309393));
#8817=CARTESIAN_POINT('Ctrl Pts',(0.065069600391363,-1.0183917429657,1.64367304400768));
#8818=CARTESIAN_POINT('Ctrl Pts',(0.031527330883376,-1.02,1.65));
#8819=CARTESIAN_POINT('Ctrl Pts',(-0.031527330883376,-1.02,1.65));
#8820=CARTESIAN_POINT('Ctrl Pts',(-0.065069600391363,-1.0183917429657,1.64367304400768));
#8821=CARTESIAN_POINT('Ctrl Pts',(-0.126627870945253,-1.01258144235289,
1.61811920309393));
#8822=CARTESIAN_POINT('Ctrl Pts',(-0.154654113568716,-1.00845756932386,
1.59889927702456));
#8823=CARTESIAN_POINT('Ctrl Pts',(-0.198902128206072,-1.00067109353237,
1.5546512623872));
#8824=CARTESIAN_POINT('Ctrl Pts',(-0.218119830014375,-0.996491737296663,
1.52662620974954));
#8825=CARTESIAN_POINT('Ctrl Pts',(-0.243672048431404,-0.990553370646674,
1.46507214966317));
#8826=CARTESIAN_POINT('Ctrl Pts',(-0.25,-0.988888264668966,1.43153139415882));
#8827=CARTESIAN_POINT('Ctrl Pts',(-0.25,-0.988888264668966,1.4));
#8828=CARTESIAN_POINT('Origin',(-1.72,2.10639249453345E-16,2.9));
#8829=CARTESIAN_POINT('',(-1.885,1.90432577267413E-16,2.9));
#8830=CARTESIAN_POINT('Origin',(-1.72,2.10639249453345E-16,2.9));
#8831=CARTESIAN_POINT('',(-1.885,2.30845921639276E-16,3.6));
#8832=CARTESIAN_POINT('',(-1.885,1.90432577267413E-16,2.9));
#8833=CARTESIAN_POINT('Origin',(-1.72,2.10639249453345E-16,3.6));
#8834=CARTESIAN_POINT('Origin',(-1.72,2.22044604925031E-16,2.9));
#8835=CARTESIAN_POINT('Origin',(1.05319624726672E-16,1.72,2.9));
#8836=CARTESIAN_POINT('',(-0.165,1.72,2.9));
#8837=CARTESIAN_POINT('Origin',(1.05319624726672E-16,1.72,2.9));
#8838=CARTESIAN_POINT('',(-0.165,1.72,3.6));
#8839=CARTESIAN_POINT('',(-0.165,1.72,2.9));
#8840=CARTESIAN_POINT('Origin',(1.05319624726672E-16,1.72,3.6));
#8841=CARTESIAN_POINT('Origin',(1.11022302462516E-16,1.72,2.9));
#8842=CARTESIAN_POINT('Origin',(1.72,0.,2.9));
#8843=CARTESIAN_POINT('',(1.555,-2.02066721859313E-17,2.9));
#8844=CARTESIAN_POINT('Origin',(1.72,0.,2.9));
#8845=CARTESIAN_POINT('',(1.555,2.02066721859313E-17,3.6));
#8846=CARTESIAN_POINT('',(1.555,-2.02066721859313E-17,2.9));
#8847=CARTESIAN_POINT('Origin',(1.72,0.,3.6));
#8848=CARTESIAN_POINT('Origin',(1.72,0.,2.9));
#8849=CARTESIAN_POINT('Origin',(-3.15958874180017E-16,-1.72,2.9));
#8850=CARTESIAN_POINT('',(-0.165,-1.72,2.9));
#8851=CARTESIAN_POINT('Origin',(-3.15958874180017E-16,-1.72,2.9));
#8852=CARTESIAN_POINT('',(-0.165,-1.72,3.6));
#8853=CARTESIAN_POINT('',(-0.165,-1.72,2.9));
#8854=CARTESIAN_POINT('Origin',(-3.15958874180017E-16,-1.72,3.6));
#8855=CARTESIAN_POINT('Origin',(-3.05311331771918E-16,-1.72,2.9));
#8856=CARTESIAN_POINT('Origin',(0.,0.,2.05));
#8857=CARTESIAN_POINT('',(-1.5,-1.83697019872103E-16,2.05));
#8858=CARTESIAN_POINT('Origin',(0.,0.,2.05));
#8859=CARTESIAN_POINT('',(-1.5,1.83697019872103E-16,3.6));
#8860=CARTESIAN_POINT('',(-1.5,-1.83697019872103E-16,2.05));
#8861=CARTESIAN_POINT('Origin',(0.,0.,3.6));
#8862=CARTESIAN_POINT('Origin',(0.,0.,2.05));
#8863=CARTESIAN_POINT('',(-1.02,-1.2491397351303E-16,2.05));
#8864=CARTESIAN_POINT('Origin',(0.,0.,2.05));
#8865=CARTESIAN_POINT('Origin',(0.,0.,0.9));
#8866=CARTESIAN_POINT('',(-1.02,-1.2491397351303E-16,1.));
#8867=CARTESIAN_POINT('Origin',(0.,0.,1.));
#8868=CARTESIAN_POINT('',(-1.02,-1.2491397351303E-16,0.9));
#8869=CARTESIAN_POINT('Origin',(5.94264068711928,-1.7,2.2));
#8870=CARTESIAN_POINT('',(6.44264068711928,-1.7,2.2));
#8871=CARTESIAN_POINT('',(6.44264068711928,-1.7,3.6));
#8872=CARTESIAN_POINT('',(6.44264068711928,-1.7,2.2));
#8873=CARTESIAN_POINT('',(5.94264068711928,-2.2,3.6));
#8874=CARTESIAN_POINT('Origin',(5.94264068711928,-1.7,3.6));
#8875=CARTESIAN_POINT('',(5.94264068711928,-2.2,2.2));
#8876=CARTESIAN_POINT('',(5.94264068711928,-2.2,2.2));
#8877=CARTESIAN_POINT('Origin',(5.94264068711928,-1.7,2.2));
#8878=CARTESIAN_POINT('Origin',(5.94264068711928,-1.7,2.2));
#8879=CARTESIAN_POINT('',(6.44264068711928,-1.7,2.2));
#8880=CARTESIAN_POINT('Origin',(5.94264068711928,-1.7,2.2));
#8881=CARTESIAN_POINT('',(5.94264068711928,-2.2,2.2));
#8882=CARTESIAN_POINT('Origin',(5.94264068711928,-1.7,3.6));
#8883=CARTESIAN_POINT('Origin',(5.94264068711928,-1.7,2.2));
#8884=CARTESIAN_POINT('',(5.66764068711928,-1.7,2.2));
#8885=CARTESIAN_POINT('Origin',(5.94264068711928,-1.7,2.2));
#8886=CARTESIAN_POINT('Origin',(-1.7,1.7,2.2));
#8887=CARTESIAN_POINT('',(-1.7,2.2,2.2));
#8888=CARTESIAN_POINT('',(-1.7,2.2,3.6));
#8889=CARTESIAN_POINT('',(-1.7,2.2,2.2));
#8890=CARTESIAN_POINT('',(-2.2,1.7,3.6));
#8891=CARTESIAN_POINT('Origin',(-1.7,1.7,3.6));
#8892=CARTESIAN_POINT('',(-2.2,1.7,2.2));
#8893=CARTESIAN_POINT('',(-2.2,1.7,2.2));
#8894=CARTESIAN_POINT('Origin',(-1.7,1.7,2.2));
#8895=CARTESIAN_POINT('Origin',(-1.7,1.7,2.2));
#8896=CARTESIAN_POINT('',(-1.7,2.2,2.2));
#8897=CARTESIAN_POINT('Origin',(-1.7,1.7,2.2));
#8898=CARTESIAN_POINT('',(-2.2,1.7,2.2));
#8899=CARTESIAN_POINT('Origin',(-1.7,1.7,3.6));
#8900=CARTESIAN_POINT('Origin',(-1.7,1.7,2.2));
#8901=CARTESIAN_POINT('',(-1.975,1.7,2.2));
#8902=CARTESIAN_POINT('Origin',(-1.7,1.7,2.2));
#8903=CARTESIAN_POINT('Origin',(-1.7,-1.7,2.2));
#8904=CARTESIAN_POINT('',(-1.7,-2.2,2.2));
#8905=CARTESIAN_POINT('',(-1.7,-2.2,3.6));
#8906=CARTESIAN_POINT('',(-1.7,-2.2,2.2));
#8907=CARTESIAN_POINT('',(-2.2,-1.7,3.6));
#8908=CARTESIAN_POINT('Origin',(-1.7,-1.7,3.6));
#8909=CARTESIAN_POINT('',(-2.2,-1.7,2.2));
#8910=CARTESIAN_POINT('',(-2.2,-1.7,2.2));
#8911=CARTESIAN_POINT('Origin',(-1.7,-1.7,2.2));
#8912=CARTESIAN_POINT('Origin',(-1.7,-1.7,2.2));
#8913=CARTESIAN_POINT('',(-1.7,-2.2,2.2));
#8914=CARTESIAN_POINT('Origin',(-1.7,-1.7,2.2));
#8915=CARTESIAN_POINT('',(-2.2,-1.7,2.2));
#8916=CARTESIAN_POINT('Origin',(-1.7,-1.7,3.6));
#8917=CARTESIAN_POINT('Origin',(-1.7,-1.7,2.2));
#8918=CARTESIAN_POINT('',(-1.975,-1.7,2.2));
#8919=CARTESIAN_POINT('Origin',(-1.7,-1.7,2.2));
#8920=CARTESIAN_POINT('Origin',(5.94264068711928,1.7,2.2));
#8921=CARTESIAN_POINT('',(5.94264068711928,2.2,2.2));
#8922=CARTESIAN_POINT('',(5.94264068711928,2.2,3.6));
#8923=CARTESIAN_POINT('',(5.94264068711928,2.2,2.2));
#8924=CARTESIAN_POINT('',(6.44264068711928,1.7,3.6));
#8925=CARTESIAN_POINT('Origin',(5.94264068711928,1.7,3.6));
#8926=CARTESIAN_POINT('',(6.44264068711928,1.7,2.2));
#8927=CARTESIAN_POINT('',(6.44264068711928,1.7,2.2));
#8928=CARTESIAN_POINT('Origin',(5.94264068711928,1.7,2.2));
#8929=CARTESIAN_POINT('Origin',(5.94264068711928,1.7,2.2));
#8930=CARTESIAN_POINT('',(5.94264068711928,2.2,2.2));
#8931=CARTESIAN_POINT('Origin',(5.94264068711928,1.7,2.2));
#8932=CARTESIAN_POINT('',(6.44264068711928,1.7,2.2));
#8933=CARTESIAN_POINT('Origin',(5.94264068711928,1.7,3.6));
#8934=CARTESIAN_POINT('Origin',(5.94264068711928,1.7,2.2));
#8935=CARTESIAN_POINT('',(5.66764068711928,1.7,2.2));
#8936=CARTESIAN_POINT('Origin',(5.94264068711928,1.7,2.2));
#8937=CARTESIAN_POINT('Origin',(2.12132034355964,0.,3.6));
#8938=CARTESIAN_POINT('',(6.44264068711929,2.2,3.6));
#8939=CARTESIAN_POINT('',(6.44264068711928,-2.2,3.6));
#8940=CARTESIAN_POINT('',(6.44264068711928,2.2,3.6));
#8941=CARTESIAN_POINT('Origin',(2.12132034355964,0.,3.6));
#8942=CARTESIAN_POINT('',(-2.2,-2.2,3.6));
#8943=CARTESIAN_POINT('',(-2.2,2.2,3.6));
#8944=CARTESIAN_POINT('',(-2.2,-2.2,3.6));
#8945=CARTESIAN_POINT('Origin',(2.12132034355964,0.,3.6));
#8946=CARTESIAN_POINT('',(-2.2,2.2,3.6));
#8947=CARTESIAN_POINT('',(6.44264068711928,2.2,3.6));
#8948=CARTESIAN_POINT('',(-2.2,2.2,3.6));
#8949=CARTESIAN_POINT('Origin',(2.12132034355964,0.,3.6));
#8950=CARTESIAN_POINT('',(6.44264068711928,-2.2,3.6));
#8951=CARTESIAN_POINT('',(6.44264068711928,2.2,3.6));
#8952=CARTESIAN_POINT('',(-2.2,2.2,3.6));
#8953=CARTESIAN_POINT('',(-2.2,-2.2,3.6));
#8954=CARTESIAN_POINT('Origin',(2.12132034355964,0.,3.6));
#8955=CARTESIAN_POINT('',(6.44264068711929,-2.2,3.6));
#8956=CARTESIAN_POINT('',(-2.2,-2.2,3.6));
#8957=CARTESIAN_POINT('',(6.44264068711928,-2.2,3.6));
#8958=CARTESIAN_POINT('Origin',(5.94264068711928,-1.7,0.9));
#8959=CARTESIAN_POINT('',(5.66764068711928,-1.7,1.));
#8960=CARTESIAN_POINT('Origin',(5.94264068711928,-1.7,1.));
#8961=CARTESIAN_POINT('',(5.66764068711928,-1.7,0.9));
#8962=CARTESIAN_POINT('Origin',(-1.7,1.7,0.9));
#8963=CARTESIAN_POINT('',(-1.975,1.7,1.));
#8964=CARTESIAN_POINT('Origin',(-1.7,1.7,1.));
#8965=CARTESIAN_POINT('',(-1.975,1.7,0.9));
#8966=CARTESIAN_POINT('Origin',(-1.7,-1.7,0.9));
#8967=CARTESIAN_POINT('',(-1.975,-1.7,1.));
#8968=CARTESIAN_POINT('Origin',(-1.7,-1.7,1.));
#8969=CARTESIAN_POINT('',(-1.975,-1.7,0.9));
#8970=CARTESIAN_POINT('Origin',(5.94264068711928,1.7,0.9));
#8971=CARTESIAN_POINT('',(5.66764068711928,1.7,1.));
#8972=CARTESIAN_POINT('Origin',(5.94264068711928,1.7,1.));
#8973=CARTESIAN_POINT('',(5.66764068711928,1.7,0.9));
#8974=CARTESIAN_POINT('Origin',(6.44264068711928,2.2,1.));
#8975=CARTESIAN_POINT('',(6.44264068711928,2.2,1.));
#8976=CARTESIAN_POINT('',(-2.2,2.2,1.));
#8977=CARTESIAN_POINT('',(6.44264068711928,2.2,1.));
#8978=CARTESIAN_POINT('',(-2.2,2.2,1.));
#8979=CARTESIAN_POINT('',(6.44264068711928,2.2,1.));
#8980=CARTESIAN_POINT('Origin',(6.44264068711928,-2.2,1.));
#8981=CARTESIAN_POINT('',(6.44264068711928,-2.2,1.));
#8982=CARTESIAN_POINT('',(6.44264068711928,-2.2,1.));
#8983=CARTESIAN_POINT('',(6.44264068711928,-2.2,1.));
#8984=CARTESIAN_POINT('Origin',(-2.2,-2.2,1.));
#8985=CARTESIAN_POINT('',(-2.2,-2.2,1.));
#8986=CARTESIAN_POINT('',(-2.2,-2.2,1.));
#8987=CARTESIAN_POINT('',(-2.2,-2.2,1.));
#8988=CARTESIAN_POINT('Origin',(-2.2,2.2,1.));
#8989=CARTESIAN_POINT('',(-2.2,2.2,1.));
#8990=CARTESIAN_POINT('Origin',(2.12132034355964,0.,1.));
#10901=UNCERTAINTY_MEASURE_WITH_UNIT(LENGTH_MEASURE(0.001),#10958,
'DISTANCE_ACCURACY_VALUE',
'Maximum model space distance between geometric entities at asserted c
onnectivities');
#10926=UNCERTAINTY_MEASURE_WITH_UNIT(LENGTH_MEASURE(0.001),#10958,
'DISTANCE_ACCURACY_VALUE',
'Maximum model space distance between geometric entities at asserted c
onnectivities');
#10932=(
GEOMETRIC_REPRESENTATION_CONTEXT(3)
GLOBAL_UNCERTAINTY_ASSIGNED_CONTEXT((#10901))
GLOBAL_UNIT_ASSIGNED_CONTEXT((#10958,#10960,#10961))
REPRESENTATION_CONTEXT('','3D')
);
#10957=(
GEOMETRIC_REPRESENTATION_CONTEXT(3)
GLOBAL_UNCERTAINTY_ASSIGNED_CONTEXT((#10926))
GLOBAL_UNIT_ASSIGNED_CONTEXT((#10958,#10960,#10961))
REPRESENTATION_CONTEXT('','3D')
);
#10958=(
LENGTH_UNIT()
NAMED_UNIT(*)
SI_UNIT(.CENTI.,.METRE.)
);
#10960=(
NAMED_UNIT(*)
PLANE_ANGLE_UNIT()
SI_UNIT($,.RADIAN.)
);
#10961=(
NAMED_UNIT(*)
SI_UNIT($,.STERADIAN.)
SOLID_ANGLE_UNIT()
);
#10967=SHAPE_DEFINITION_REPRESENTATION(#10997,#11069);
#10997=PRODUCT_DEFINITION_SHAPE('',$,#11100);
#11069=SHAPE_REPRESENTATION('',(#6045),#10932);
#11094=PRODUCT_DEFINITION_CONTEXT('part definition',#11186,'design');
#11100=PRODUCT_DEFINITION('Twin bearing block','Twin bearing block',#11130,
#11094);
#11130=PRODUCT_DEFINITION_FORMATION('',$,#11193);
#11186=APPLICATION_CONTEXT(
'Core Data for Automotive Mechanical Design Process');
#11187=PRODUCT_CONTEXT('part definition',#11186,'mechanical');
#11193=PRODUCT('Twin bearing block','Twin bearing block',
'Twin bearing block',(#11187));
#11281=COLOUR_RGB('Grey',0.48,0.52,0.57);
#11282=FILL_AREA_STYLE_COLOUR('',#11281);
#11283=FILL_AREA_STYLE('',(#11282));
#11284=SURFACE_STYLE_FILL_AREA(#11283);
#11285=SURFACE_SIDE_STYLE('',(#11284));
#11286=SURFACE_STYLE_USAGE(.BOTH.,#11285);
#11287=PRESENTATION_STYLE_ASSIGNMENT((#11286));
ENDSEC;
END-ISO-10303-21;
